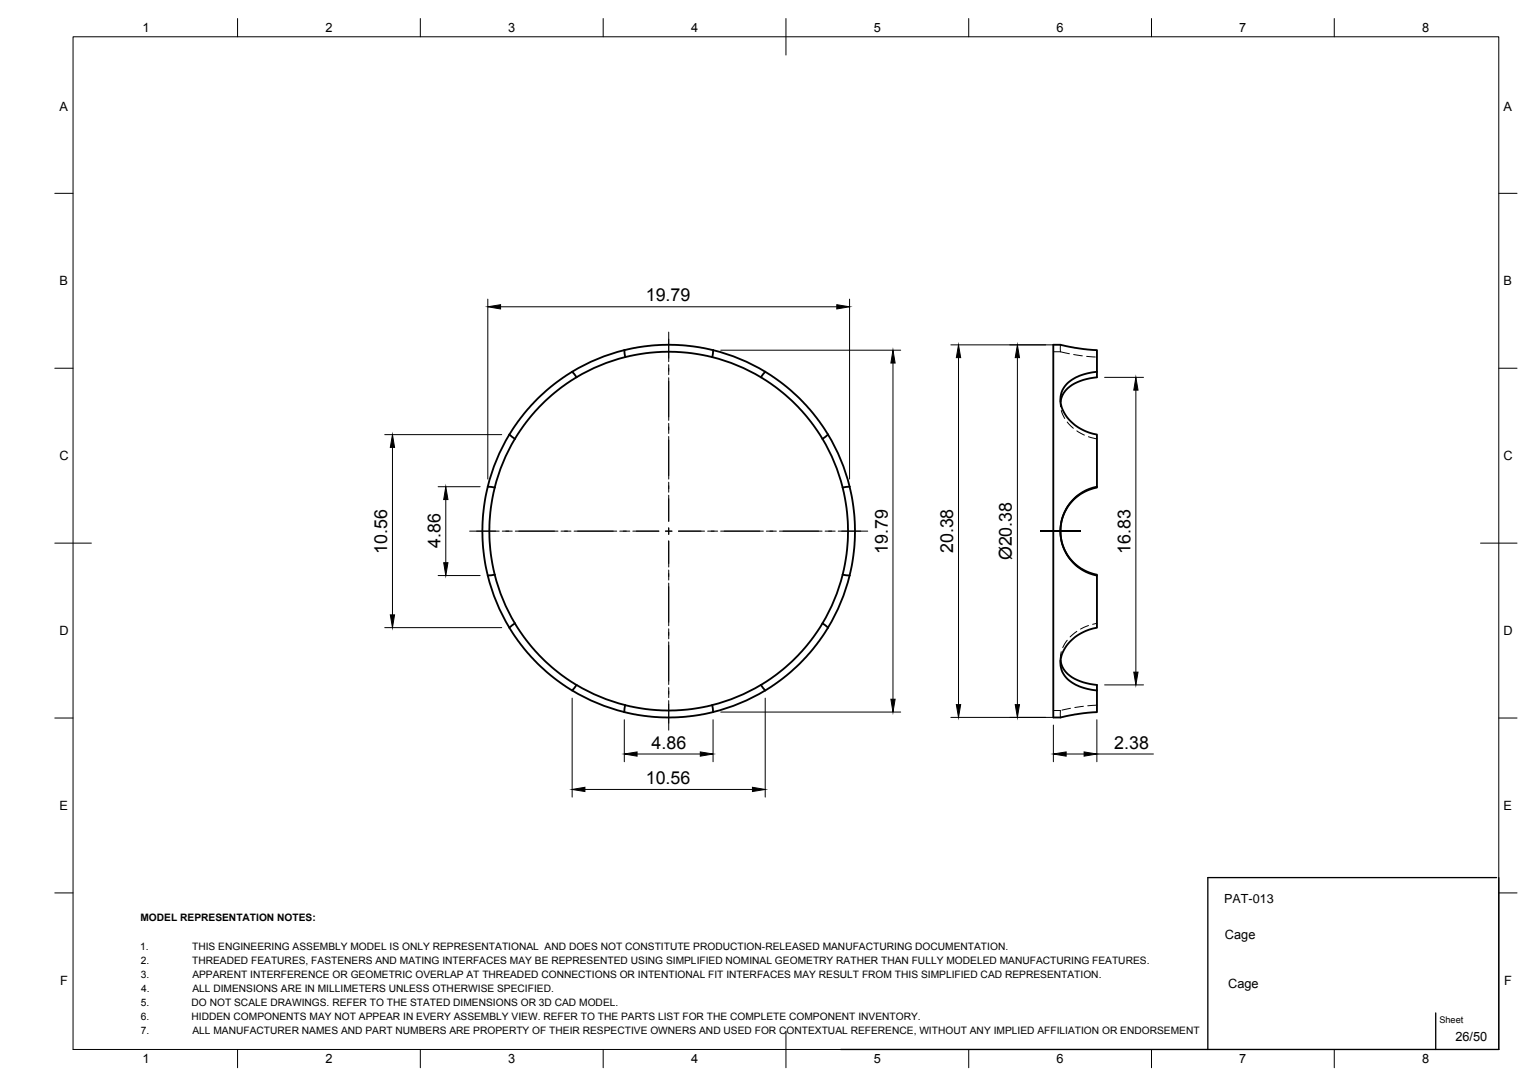
ISO-10303-21;
HEADER;
/* Generated by software containing ST-Developer
 * from STEP Tools, Inc. (www.steptools.com) 
 */

FILE_DESCRIPTION(
/* description */ ('Belt-driven linear axis on 2020 extrusion'),
/* implementation_level */ '2;1');

FILE_NAME(
/* name */ 'Cage.step',
/* time_stamp */ '2026-10-28T03:26:09-07:00',
/* author */ (''),
/* organization */ (''),
/* preprocessor_version */ 'ST-DEVELOPER v20.2',
/* originating_system */ 'Autodesk Translation Framework v15.17.0.0',
/* authorisation */ '');

FILE_SCHEMA (('AUTOMOTIVE_DESIGN { 1 0 10303 214 3 1 1 }'));
ENDSEC;

DATA;
#10=MECHANICAL_DESIGN_GEOMETRIC_PRESENTATION_REPRESENTATION('',(#636),#20096);
#441=B_SPLINE_CURVE_WITH_KNOTS('',3,(#17380,#17381,#17382,#17383,#17384,
#17385,#17386,#17387,#17388,#17389,#17390,#17391,#17392,#17393,#17394,#17395,
#17396,#17397,#17398,#17399,#17400,#17401),.UNSPECIFIED.,.F.,.F.,(4,2,2,
2,2,2,2,2,2,2,4),(0.0473477652366656,0.126350602536658,0.189525903804987,
0.252701205073317,0.313298422430275,0.373895639787233,0.434492857144191,
0.495090074501149,0.558265375769478,0.621440677037807,0.7004435143378),
 .UNSPECIFIED.);
#442=B_SPLINE_CURVE_WITH_KNOTS('',3,(#17405,#17406,#17407,#17408,#17409,
#17410,#17411,#17412,#17413,#17414,#17415,#17416,#17417,#17418,#17419,#17420,
#17421,#17422,#17423,#17424,#17425,#17426),.UNSPECIFIED.,.F.,.F.,(4,2,2,
2,2,2,2,2,2,2,4),(0.0464897534940957,0.0852567806515119,0.170513561303024,
0.246687263103517,0.308657850341199,0.370628437578881,0.432599024816563,
0.494569612054245,0.570743313854739,0.656000094506251,0.694767121663666),
 .UNSPECIFIED.);
#443=B_SPLINE_CURVE_WITH_KNOTS('',3,(#17432,#17433,#17434,#17435,#17436,
#17437,#17438,#17439,#17440,#17441,#17442,#17443,#17444,#17445,#17446,#17447,
#17448,#17449,#17450,#17451,#17452,#17453),.UNSPECIFIED.,.F.,.F.,(4,2,2,
2,2,2,2,2,2,2,4),(0.0464897534940957,0.0852567806515118,0.170513561303024,
0.246687263103517,0.308657850341199,0.370628437578881,0.432599024816563,
0.494569612054245,0.570743313854738,0.65600009450625,0.694767121663666),
 .UNSPECIFIED.);
#444=B_SPLINE_CURVE_WITH_KNOTS('',3,(#17457,#17458,#17459,#17460,#17461,
#17462,#17463,#17464,#17465,#17466,#17467,#17468,#17469,#17470,#17471,#17472,
#17473,#17474,#17475,#17476,#17477,#17478),.UNSPECIFIED.,.F.,.F.,(4,2,2,
2,2,2,2,2,2,2,4),(0.0464897534940957,0.0852567806515119,0.170513561303024,
0.246687263103517,0.308657850341199,0.370628437578881,0.432599024816563,
0.494569612054245,0.570743313854739,0.656000094506251,0.694767121663666),
 .UNSPECIFIED.);
#445=B_SPLINE_CURVE_WITH_KNOTS('',3,(#17482,#17483,#17484,#17485,#17486,
#17487,#17488,#17489,#17490,#17491,#17492,#17493),.UNSPECIFIED.,.F.,.F.,
(4,2,2,2,2,4),(0.0464897534940957,0.0852567806515119,0.170513561303024,
0.246687263103517,0.308657850341199,0.370628437578881),.UNSPECIFIED.);
#446=B_SPLINE_CURVE_WITH_KNOTS('',3,(#17498,#17499,#17500,#17501,#17502,
#17503,#17504,#17505,#17506,#17507,#17508,#17509),.UNSPECIFIED.,.F.,.F.,
(4,2,2,2,2,4),(0.370628437578881,0.432599024816563,0.494569612054245,0.570743313854738,
0.65600009450625,0.694767121663666),.UNSPECIFIED.);
#447=B_SPLINE_CURVE_WITH_KNOTS('',3,(#17513,#17514,#17515,#17516,#17517,
#17518,#17519,#17520,#17521,#17522,#17523,#17524,#17525,#17526,#17527,#17528,
#17529,#17530,#17531,#17532,#17533,#17534),.UNSPECIFIED.,.F.,.F.,(4,2,2,
2,2,2,2,2,2,2,4),(0.0464897534940957,0.0852567806515121,0.170513561303024,
0.246687263103518,0.308657850341199,0.370628437578881,0.432599024816563,
0.494569612054245,0.570743313854738,0.65600009450625,0.694767121663666),
 .UNSPECIFIED.);
#448=B_SPLINE_CURVE_WITH_KNOTS('',3,(#17538,#17539,#17540,#17541,#17542,
#17543,#17544,#17545,#17546,#17547,#17548,#17549,#17550,#17551,#17552,#17553,
#17554,#17555,#17556,#17557,#17558,#17559),.UNSPECIFIED.,.F.,.F.,(4,2,2,
2,2,2,2,2,2,2,4),(0.0464897534940957,0.0852567806515119,0.170513561303024,
0.246687263103517,0.308657850341199,0.370628437578881,0.432599024816563,
0.494569612054245,0.570743313854738,0.65600009450625,0.694767121663667),
 .UNSPECIFIED.);
#449=B_SPLINE_CURVE_WITH_KNOTS('',3,(#17563,#17564,#17565,#17566,#17567,
#17568,#17569,#17570,#17571,#17572,#17573,#17574,#17575,#17576,#17577,#17578,
#17579,#17580,#17581,#17582,#17583,#17584),.UNSPECIFIED.,.F.,.F.,(4,2,2,
2,2,2,2,2,2,2,4),(0.0464897534940957,0.0852567806515119,0.170513561303024,
0.246687263103517,0.308657850341199,0.370628437578881,0.432599024816563,
0.494569612054245,0.570743313854738,0.65600009450625,0.694767121663666),
 .UNSPECIFIED.);
#450=B_SPLINE_CURVE_WITH_KNOTS('',3,(#17588,#17589,#17590,#17591,#17592,
#17593,#17594,#17595,#17596,#17597,#17598,#17599,#17600,#17601,#17602,#17603,
#17604,#17605,#17606,#17607,#17608,#17609),.UNSPECIFIED.,.F.,.F.,(4,2,2,
2,2,2,2,2,2,2,4),(0.0464897534940957,0.0852567806515119,0.170513561303024,
0.246687263103517,0.308657850341199,0.370628437578881,0.432599024816563,
0.494569612054245,0.570743313854739,0.656000094506251,0.694767121663667),
 .UNSPECIFIED.);
#451=B_SPLINE_CURVE_WITH_KNOTS('',3,(#17617,#17618,#17619,#17620,#17621,
#17622,#17623,#17624,#17625,#17626,#17627,#17628,#17629,#17630,#17631,#17632,
#17633,#17634,#17635,#17636,#17637,#17638),.UNSPECIFIED.,.F.,.F.,(4,2,2,
2,2,2,2,2,2,2,4),(0.0473477652366656,0.126350602536658,0.189525903804987,
0.252701205073316,0.313298422430274,0.373895639787232,0.434492857144191,
0.495090074501149,0.558265375769478,0.621440677037807,0.7004435143378),
 .UNSPECIFIED.);
#452=B_SPLINE_CURVE_WITH_KNOTS('',3,(#17646,#17647,#17648,#17649,#17650,
#17651,#17652,#17653,#17654,#17655,#17656,#17657,#17658,#17659,#17660,#17661,
#17662,#17663,#17664,#17665,#17666,#17667),.UNSPECIFIED.,.F.,.F.,(4,2,2,
2,2,2,2,2,2,2,4),(0.0473477652366656,0.126350602536658,0.189525903804987,
0.252701205073317,0.313298422430275,0.373895639787233,0.434492857144191,
0.495090074501149,0.558265375769478,0.621440677037807,0.7004435143378),
 .UNSPECIFIED.);
#453=B_SPLINE_CURVE_WITH_KNOTS('',3,(#17676,#17677,#17678,#17679,#17680,
#17681,#17682,#17683,#17684,#17685,#17686,#17687),.UNSPECIFIED.,.F.,.F.,
(4,2,2,2,2,4),(0.0473477652366656,0.126350602536658,0.189525903804987,0.252701205073316,
0.313298422430275,0.373895639787233),.UNSPECIFIED.);
#454=B_SPLINE_CURVE_WITH_KNOTS('',3,(#17689,#17690,#17691,#17692,#17693,
#17694,#17695,#17696,#17697,#17698,#17699,#17700),.UNSPECIFIED.,.F.,.F.,
(4,2,2,2,2,4),(0.373895639787233,0.434492857144191,0.495090074501149,0.558265375769478,
0.621440677037807,0.7004435143378),.UNSPECIFIED.);
#455=B_SPLINE_CURVE_WITH_KNOTS('',3,(#17707,#17708,#17709,#17710,#17711,
#17712,#17713,#17714,#17715,#17716,#17717,#17718,#17719,#17720,#17721,#17722,
#17723,#17724,#17725,#17726,#17727,#17728),.UNSPECIFIED.,.F.,.F.,(4,2,2,
2,2,2,2,2,2,2,4),(0.0473477652366656,0.126350602536658,0.189525903804987,
0.252701205073316,0.313298422430275,0.373895639787233,0.434492857144191,
0.495090074501149,0.558265375769478,0.621440677037807,0.7004435143378),
 .UNSPECIFIED.);
#456=B_SPLINE_CURVE_WITH_KNOTS('',3,(#17736,#17737,#17738,#17739,#17740,
#17741,#17742,#17743,#17744,#17745,#17746,#17747,#17748,#17749,#17750,#17751,
#17752,#17753,#17754,#17755,#17756,#17757),.UNSPECIFIED.,.F.,.F.,(4,2,2,
2,2,2,2,2,2,2,4),(0.0473477652366656,0.126350602536658,0.189525903804987,
0.252701205073317,0.313298422430275,0.373895639787233,0.434492857144191,
0.495090074501149,0.558265375769478,0.621440677037807,0.7004435143378),
 .UNSPECIFIED.);
#457=B_SPLINE_CURVE_WITH_KNOTS('',3,(#17765,#17766,#17767,#17768,#17769,
#17770,#17771,#17772,#17773,#17774,#17775,#17776,#17777,#17778,#17779,#17780,
#17781,#17782,#17783,#17784,#17785,#17786),.UNSPECIFIED.,.F.,.F.,(4,2,2,
2,2,2,2,2,2,2,4),(0.0473477652366656,0.126350602536658,0.189525903804987,
0.252701205073316,0.313298422430275,0.373895639787233,0.434492857144191,
0.495090074501149,0.558265375769478,0.621440677037807,0.7004435143378),
 .UNSPECIFIED.);
#458=B_SPLINE_CURVE_WITH_KNOTS('',3,(#17795,#17796,#17797,#17798,#17799,
#17800,#17801,#17802,#17803,#17804,#17805,#17806,#17807,#17808,#17809,#17810,
#17811,#17812,#17813,#17814,#17815,#17816),.UNSPECIFIED.,.F.,.F.,(4,2,2,
2,2,2,2,2,2,2,4),(0.0473477652366656,0.126350602536658,0.189525903804987,
0.252701205073317,0.313298422430275,0.373895639787233,0.434492857144191,
0.495090074501149,0.558265375769478,0.621440677037807,0.7004435143378),
 .UNSPECIFIED.);
#489=SPHERICAL_SURFACE('',#11975,0.247676);
#490=SPHERICAL_SURFACE('',#11991,0.247676);
#491=SPHERICAL_SURFACE('',#11996,0.247676);
#492=SPHERICAL_SURFACE('',#12001,0.247676);
#493=SPHERICAL_SURFACE('',#12006,0.247676);
#494=SPHERICAL_SURFACE('',#12011,0.247676);
#495=SPHERICAL_SURFACE('',#12016,0.247676);
#496=SPHERICAL_SURFACE('',#12024,0.247676);
#535=SHAPE_REPRESENTATION_RELATIONSHIP('SRR','None',#20332,#581);
#581=ADVANCED_BREP_SHAPE_REPRESENTATION('',(#692),#20063);
#636=STYLED_ITEM('',(#20650),#692);
#692=MANIFOLD_SOLID_BREP('Continuous crown cage',#10949);
#808=FACE_BOUND('',#2218,.T.);
#1009=PLANE('',#11988);
#1010=PLANE('',#11993);
#1011=PLANE('',#11998);
#1012=PLANE('',#12003);
#1013=PLANE('',#12008);
#1014=PLANE('',#12013);
#1015=PLANE('',#12022);
#1016=PLANE('',#12026);
#1017=PLANE('',#12027);
#1488=FACE_OUTER_BOUND('',#2200,.T.);
#1489=FACE_OUTER_BOUND('',#2201,.T.);
#1490=FACE_OUTER_BOUND('',#2202,.T.);
#1491=FACE_OUTER_BOUND('',#2203,.T.);
#1492=FACE_OUTER_BOUND('',#2204,.T.);
#1493=FACE_OUTER_BOUND('',#2205,.T.);
#1494=FACE_OUTER_BOUND('',#2206,.T.);
#1495=FACE_OUTER_BOUND('',#2207,.T.);
#1496=FACE_OUTER_BOUND('',#2208,.T.);
#1497=FACE_OUTER_BOUND('',#2209,.T.);
#1498=FACE_OUTER_BOUND('',#2210,.T.);
#1499=FACE_OUTER_BOUND('',#2211,.T.);
#1500=FACE_OUTER_BOUND('',#2212,.T.);
#1501=FACE_OUTER_BOUND('',#2213,.T.);
#1502=FACE_OUTER_BOUND('',#2214,.T.);
#1503=FACE_OUTER_BOUND('',#2215,.T.);
#1504=FACE_OUTER_BOUND('',#2216,.T.);
#1505=FACE_OUTER_BOUND('',#2217,.T.);
#1506=FACE_OUTER_BOUND('',#2219,.T.);
#2200=EDGE_LOOP('',(#8305,#8306,#8307,#8308));
#2201=EDGE_LOOP('',(#8309,#8310,#8311,#8312,#8313,#8314,#8315,#8316,#8317,
#8318,#8319,#8320,#8321,#8322,#8323,#8324,#8325,#8326,#8327,#8328));
#2202=EDGE_LOOP('',(#8329,#8330,#8331,#8332));
#2203=EDGE_LOOP('',(#8333,#8334,#8335,#8336));
#2204=EDGE_LOOP('',(#8337,#8338,#8339,#8340));
#2205=EDGE_LOOP('',(#8341,#8342,#8343,#8344));
#2206=EDGE_LOOP('',(#8345,#8346,#8347,#8348));
#2207=EDGE_LOOP('',(#8349,#8350,#8351,#8352,#8353,#8354));
#2208=EDGE_LOOP('',(#8355,#8356,#8357,#8358));
#2209=EDGE_LOOP('',(#8359,#8360,#8361,#8362));
#2210=EDGE_LOOP('',(#8363,#8364,#8365,#8366));
#2211=EDGE_LOOP('',(#8367,#8368,#8369,#8370));
#2212=EDGE_LOOP('',(#8371,#8372,#8373,#8374));
#2213=EDGE_LOOP('',(#8375,#8376,#8377,#8378));
#2214=EDGE_LOOP('',(#8379,#8380,#8381,#8382,#8383,#8384,#8385,#8386,#8387,
#8388,#8389,#8390,#8391,#8392,#8393,#8394,#8395,#8396,#8397,#8398));
#2215=EDGE_LOOP('',(#8399,#8400,#8401,#8402));
#2216=EDGE_LOOP('',(#8403,#8404,#8405,#8406));
#2217=EDGE_LOOP('',(#8407));
#2218=EDGE_LOOP('',(#8408));
#2219=EDGE_LOOP('',(#8409,#8410,#8411,#8412));
#2965=LINE('',#17495,#3822);
#2966=LINE('',#17791,#3823);
#3822=VECTOR('',#14069,1.019052);
#3823=VECTOR('',#14146,0.980948);
#4605=CIRCLE('',#11976,0.243053047864041);
#4606=CIRCLE('',#11977,0.243053047864041);
#4607=CIRCLE('',#11979,1.019052);
#4608=CIRCLE('',#11980,1.019052);
#4609=CIRCLE('',#11981,1.019052);
#4610=CIRCLE('',#11982,1.019052);
#4611=CIRCLE('',#11983,1.019052);
#4612=CIRCLE('',#11984,1.019052);
#4613=CIRCLE('',#11985,1.019052);
#4614=CIRCLE('',#11986,1.019052);
#4615=CIRCLE('',#11987,1.019052);
#4616=CIRCLE('',#11989,0.980948);
#4617=CIRCLE('',#11990,0.243053047864041);
#4618=CIRCLE('',#11992,0.243053047864041);
#4619=CIRCLE('',#11994,0.980948);
#4620=CIRCLE('',#11995,0.243053047864041);
#4621=CIRCLE('',#11997,0.243053047864041);
#4622=CIRCLE('',#11999,0.980948);
#4623=CIRCLE('',#12000,0.243053047864041);
#4624=CIRCLE('',#12002,0.243053047864041);
#4625=CIRCLE('',#12004,0.980948);
#4626=CIRCLE('',#12005,0.243053047864041);
#4627=CIRCLE('',#12007,0.243053047864041);
#4628=CIRCLE('',#12009,0.980948);
#4629=CIRCLE('',#12010,0.243053047864041);
#4630=CIRCLE('',#12012,0.243053047864041);
#4631=CIRCLE('',#12014,0.980948);
#4632=CIRCLE('',#12015,0.243053047864041);
#4633=CIRCLE('',#12017,0.243053047864041);
#4634=CIRCLE('',#12019,0.980948);
#4635=CIRCLE('',#12020,0.980948);
#4636=CIRCLE('',#12021,0.980948);
#4637=CIRCLE('',#12023,0.243053047864041);
#4638=CIRCLE('',#12025,0.243053047864041);
#5252=VERTEX_POINT('',#17378);
#5253=VERTEX_POINT('',#17379);
#5254=VERTEX_POINT('',#17402);
#5255=VERTEX_POINT('',#17404);
#5256=VERTEX_POINT('',#17429);
#5257=VERTEX_POINT('',#17431);
#5258=VERTEX_POINT('',#17454);
#5259=VERTEX_POINT('',#17456);
#5260=VERTEX_POINT('',#17479);
#5261=VERTEX_POINT('',#17481);
#5262=VERTEX_POINT('',#17494);
#5263=VERTEX_POINT('',#17497);
#5264=VERTEX_POINT('',#17510);
#5265=VERTEX_POINT('',#17512);
#5266=VERTEX_POINT('',#17535);
#5267=VERTEX_POINT('',#17537);
#5268=VERTEX_POINT('',#17560);
#5269=VERTEX_POINT('',#17562);
#5270=VERTEX_POINT('',#17585);
#5271=VERTEX_POINT('',#17587);
#5272=VERTEX_POINT('',#17612);
#5273=VERTEX_POINT('',#17616);
#5274=VERTEX_POINT('',#17641);
#5275=VERTEX_POINT('',#17645);
#5276=VERTEX_POINT('',#17670);
#5277=VERTEX_POINT('',#17674);
#5278=VERTEX_POINT('',#17675);
#5279=VERTEX_POINT('',#17702);
#5280=VERTEX_POINT('',#17706);
#5281=VERTEX_POINT('',#17731);
#5282=VERTEX_POINT('',#17735);
#5283=VERTEX_POINT('',#17760);
#5284=VERTEX_POINT('',#17764);
#5285=VERTEX_POINT('',#17789);
#5286=VERTEX_POINT('',#17792);
#5287=VERTEX_POINT('',#17794);
#6367=EDGE_CURVE('',#5252,#5253,#441,.T.);
#6368=EDGE_CURVE('',#5254,#5252,#4605,.T.);
#6369=EDGE_CURVE('',#5255,#5254,#442,.T.);
#6370=EDGE_CURVE('',#5253,#5255,#4606,.T.);
#6371=EDGE_CURVE('',#5256,#5254,#4607,.T.);
#6372=EDGE_CURVE('',#5256,#5257,#443,.T.);
#6373=EDGE_CURVE('',#5258,#5257,#4608,.T.);
#6374=EDGE_CURVE('',#5258,#5259,#444,.T.);
#6375=EDGE_CURVE('',#5260,#5259,#4609,.T.);
#6376=EDGE_CURVE('',#5260,#5261,#445,.T.);
#6377=EDGE_CURVE('',#5261,#5262,#2965,.T.);
#6378=EDGE_CURVE('',#5262,#5262,#4610,.T.);
#6379=EDGE_CURVE('',#5261,#5263,#446,.T.);
#6380=EDGE_CURVE('',#5264,#5263,#4611,.T.);
#6381=EDGE_CURVE('',#5264,#5265,#447,.T.);
#6382=EDGE_CURVE('',#5266,#5265,#4612,.T.);
#6383=EDGE_CURVE('',#5266,#5267,#448,.T.);
#6384=EDGE_CURVE('',#5268,#5267,#4613,.T.);
#6385=EDGE_CURVE('',#5268,#5269,#449,.T.);
#6386=EDGE_CURVE('',#5270,#5269,#4614,.T.);
#6387=EDGE_CURVE('',#5270,#5271,#450,.T.);
#6388=EDGE_CURVE('',#5255,#5271,#4615,.T.);
#6389=EDGE_CURVE('',#5252,#5272,#4616,.T.);
#6390=EDGE_CURVE('',#5272,#5256,#4617,.T.);
#6391=EDGE_CURVE('',#5273,#5272,#451,.T.);
#6392=EDGE_CURVE('',#5257,#5273,#4618,.T.);
#6393=EDGE_CURVE('',#5273,#5274,#4619,.T.);
#6394=EDGE_CURVE('',#5274,#5258,#4620,.T.);
#6395=EDGE_CURVE('',#5275,#5274,#452,.T.);
#6396=EDGE_CURVE('',#5259,#5275,#4621,.T.);
#6397=EDGE_CURVE('',#5275,#5276,#4622,.T.);
#6398=EDGE_CURVE('',#5276,#5260,#4623,.T.);
#6399=EDGE_CURVE('',#5277,#5278,#453,.T.);
#6400=EDGE_CURVE('',#5263,#5277,#4624,.T.);
#6401=EDGE_CURVE('',#5278,#5276,#454,.T.);
#6402=EDGE_CURVE('',#5277,#5279,#4625,.T.);
#6403=EDGE_CURVE('',#5279,#5264,#4626,.T.);
#6404=EDGE_CURVE('',#5280,#5279,#455,.T.);
#6405=EDGE_CURVE('',#5265,#5280,#4627,.T.);
#6406=EDGE_CURVE('',#5280,#5281,#4628,.T.);
#6407=EDGE_CURVE('',#5281,#5266,#4629,.T.);
#6408=EDGE_CURVE('',#5282,#5281,#456,.T.);
#6409=EDGE_CURVE('',#5267,#5282,#4630,.T.);
#6410=EDGE_CURVE('',#5282,#5283,#4631,.T.);
#6411=EDGE_CURVE('',#5283,#5268,#4632,.T.);
#6412=EDGE_CURVE('',#5284,#5283,#457,.T.);
#6413=EDGE_CURVE('',#5269,#5284,#4633,.T.);
#6414=EDGE_CURVE('',#5285,#5285,#4634,.T.);
#6415=EDGE_CURVE('',#5285,#5278,#2966,.T.);
#6416=EDGE_CURVE('',#5286,#5253,#4635,.T.);
#6417=EDGE_CURVE('',#5286,#5287,#458,.T.);
#6418=EDGE_CURVE('',#5284,#5287,#4636,.T.);
#6419=EDGE_CURVE('',#5271,#5286,#4637,.T.);
#6420=EDGE_CURVE('',#5287,#5270,#4638,.T.);
#8305=ORIENTED_EDGE('',*,*,#6367,.F.);
#8306=ORIENTED_EDGE('',*,*,#6368,.F.);
#8307=ORIENTED_EDGE('',*,*,#6369,.F.);
#8308=ORIENTED_EDGE('',*,*,#6370,.F.);
#8309=ORIENTED_EDGE('',*,*,#6369,.T.);
#8310=ORIENTED_EDGE('',*,*,#6371,.F.);
#8311=ORIENTED_EDGE('',*,*,#6372,.T.);
#8312=ORIENTED_EDGE('',*,*,#6373,.F.);
#8313=ORIENTED_EDGE('',*,*,#6374,.T.);
#8314=ORIENTED_EDGE('',*,*,#6375,.F.);
#8315=ORIENTED_EDGE('',*,*,#6376,.T.);
#8316=ORIENTED_EDGE('',*,*,#6377,.T.);
#8317=ORIENTED_EDGE('',*,*,#6378,.F.);
#8318=ORIENTED_EDGE('',*,*,#6377,.F.);
#8319=ORIENTED_EDGE('',*,*,#6379,.T.);
#8320=ORIENTED_EDGE('',*,*,#6380,.F.);
#8321=ORIENTED_EDGE('',*,*,#6381,.T.);
#8322=ORIENTED_EDGE('',*,*,#6382,.F.);
#8323=ORIENTED_EDGE('',*,*,#6383,.T.);
#8324=ORIENTED_EDGE('',*,*,#6384,.F.);
#8325=ORIENTED_EDGE('',*,*,#6385,.T.);
#8326=ORIENTED_EDGE('',*,*,#6386,.F.);
#8327=ORIENTED_EDGE('',*,*,#6387,.T.);
#8328=ORIENTED_EDGE('',*,*,#6388,.F.);
#8329=ORIENTED_EDGE('',*,*,#6368,.T.);
#8330=ORIENTED_EDGE('',*,*,#6389,.T.);
#8331=ORIENTED_EDGE('',*,*,#6390,.T.);
#8332=ORIENTED_EDGE('',*,*,#6371,.T.);
#8333=ORIENTED_EDGE('',*,*,#6391,.F.);
#8334=ORIENTED_EDGE('',*,*,#6392,.F.);
#8335=ORIENTED_EDGE('',*,*,#6372,.F.);
#8336=ORIENTED_EDGE('',*,*,#6390,.F.);
#8337=ORIENTED_EDGE('',*,*,#6392,.T.);
#8338=ORIENTED_EDGE('',*,*,#6393,.T.);
#8339=ORIENTED_EDGE('',*,*,#6394,.T.);
#8340=ORIENTED_EDGE('',*,*,#6373,.T.);
#8341=ORIENTED_EDGE('',*,*,#6395,.F.);
#8342=ORIENTED_EDGE('',*,*,#6396,.F.);
#8343=ORIENTED_EDGE('',*,*,#6374,.F.);
#8344=ORIENTED_EDGE('',*,*,#6394,.F.);
#8345=ORIENTED_EDGE('',*,*,#6396,.T.);
#8346=ORIENTED_EDGE('',*,*,#6397,.T.);
#8347=ORIENTED_EDGE('',*,*,#6398,.T.);
#8348=ORIENTED_EDGE('',*,*,#6375,.T.);
#8349=ORIENTED_EDGE('',*,*,#6399,.F.);
#8350=ORIENTED_EDGE('',*,*,#6400,.F.);
#8351=ORIENTED_EDGE('',*,*,#6379,.F.);
#8352=ORIENTED_EDGE('',*,*,#6376,.F.);
#8353=ORIENTED_EDGE('',*,*,#6398,.F.);
#8354=ORIENTED_EDGE('',*,*,#6401,.F.);
#8355=ORIENTED_EDGE('',*,*,#6400,.T.);
#8356=ORIENTED_EDGE('',*,*,#6402,.T.);
#8357=ORIENTED_EDGE('',*,*,#6403,.T.);
#8358=ORIENTED_EDGE('',*,*,#6380,.T.);
#8359=ORIENTED_EDGE('',*,*,#6404,.F.);
#8360=ORIENTED_EDGE('',*,*,#6405,.F.);
#8361=ORIENTED_EDGE('',*,*,#6381,.F.);
#8362=ORIENTED_EDGE('',*,*,#6403,.F.);
#8363=ORIENTED_EDGE('',*,*,#6405,.T.);
#8364=ORIENTED_EDGE('',*,*,#6406,.T.);
#8365=ORIENTED_EDGE('',*,*,#6407,.T.);
#8366=ORIENTED_EDGE('',*,*,#6382,.T.);
#8367=ORIENTED_EDGE('',*,*,#6408,.F.);
#8368=ORIENTED_EDGE('',*,*,#6409,.F.);
#8369=ORIENTED_EDGE('',*,*,#6383,.F.);
#8370=ORIENTED_EDGE('',*,*,#6407,.F.);
#8371=ORIENTED_EDGE('',*,*,#6409,.T.);
#8372=ORIENTED_EDGE('',*,*,#6410,.T.);
#8373=ORIENTED_EDGE('',*,*,#6411,.T.);
#8374=ORIENTED_EDGE('',*,*,#6384,.T.);
#8375=ORIENTED_EDGE('',*,*,#6385,.F.);
#8376=ORIENTED_EDGE('',*,*,#6411,.F.);
#8377=ORIENTED_EDGE('',*,*,#6412,.F.);
#8378=ORIENTED_EDGE('',*,*,#6413,.F.);
#8379=ORIENTED_EDGE('',*,*,#6414,.F.);
#8380=ORIENTED_EDGE('',*,*,#6415,.T.);
#8381=ORIENTED_EDGE('',*,*,#6401,.T.);
#8382=ORIENTED_EDGE('',*,*,#6397,.F.);
#8383=ORIENTED_EDGE('',*,*,#6395,.T.);
#8384=ORIENTED_EDGE('',*,*,#6393,.F.);
#8385=ORIENTED_EDGE('',*,*,#6391,.T.);
#8386=ORIENTED_EDGE('',*,*,#6389,.F.);
#8387=ORIENTED_EDGE('',*,*,#6367,.T.);
#8388=ORIENTED_EDGE('',*,*,#6416,.F.);
#8389=ORIENTED_EDGE('',*,*,#6417,.T.);
#8390=ORIENTED_EDGE('',*,*,#6418,.F.);
#8391=ORIENTED_EDGE('',*,*,#6412,.T.);
#8392=ORIENTED_EDGE('',*,*,#6410,.F.);
#8393=ORIENTED_EDGE('',*,*,#6408,.T.);
#8394=ORIENTED_EDGE('',*,*,#6406,.F.);
#8395=ORIENTED_EDGE('',*,*,#6404,.T.);
#8396=ORIENTED_EDGE('',*,*,#6402,.F.);
#8397=ORIENTED_EDGE('',*,*,#6399,.T.);
#8398=ORIENTED_EDGE('',*,*,#6415,.F.);
#8399=ORIENTED_EDGE('',*,*,#6370,.T.);
#8400=ORIENTED_EDGE('',*,*,#6388,.T.);
#8401=ORIENTED_EDGE('',*,*,#6419,.T.);
#8402=ORIENTED_EDGE('',*,*,#6416,.T.);
#8403=ORIENTED_EDGE('',*,*,#6387,.F.);
#8404=ORIENTED_EDGE('',*,*,#6420,.F.);
#8405=ORIENTED_EDGE('',*,*,#6417,.F.);
#8406=ORIENTED_EDGE('',*,*,#6419,.F.);
#8407=ORIENTED_EDGE('',*,*,#6378,.T.);
#8408=ORIENTED_EDGE('',*,*,#6414,.T.);
#8409=ORIENTED_EDGE('',*,*,#6413,.T.);
#8410=ORIENTED_EDGE('',*,*,#6418,.T.);
#8411=ORIENTED_EDGE('',*,*,#6420,.T.);
#8412=ORIENTED_EDGE('',*,*,#6386,.T.);
#10181=CYLINDRICAL_SURFACE('',#11978,1.019052);
#10182=CYLINDRICAL_SURFACE('',#12018,0.980948);
#10539=ADVANCED_FACE('',(#1488),#489,.F.);
#10540=ADVANCED_FACE('',(#1489),#10181,.T.);
#10541=ADVANCED_FACE('',(#1490),#1009,.T.);
#10542=ADVANCED_FACE('',(#1491),#490,.F.);
#10543=ADVANCED_FACE('',(#1492),#1010,.T.);
#10544=ADVANCED_FACE('',(#1493),#491,.F.);
#10545=ADVANCED_FACE('',(#1494),#1011,.T.);
#10546=ADVANCED_FACE('',(#1495),#492,.F.);
#10547=ADVANCED_FACE('',(#1496),#1012,.T.);
#10548=ADVANCED_FACE('',(#1497),#493,.F.);
#10549=ADVANCED_FACE('',(#1498),#1013,.T.);
#10550=ADVANCED_FACE('',(#1499),#494,.F.);
#10551=ADVANCED_FACE('',(#1500),#1014,.T.);
#10552=ADVANCED_FACE('',(#1501),#495,.F.);
#10553=ADVANCED_FACE('',(#1502),#10182,.F.);
#10554=ADVANCED_FACE('',(#1503),#1015,.T.);
#10555=ADVANCED_FACE('',(#1504),#496,.F.);
#10556=ADVANCED_FACE('',(#1505,#808),#1016,.T.);
#10557=ADVANCED_FACE('',(#1506),#1017,.T.);
#10949=CLOSED_SHELL('',(#10539,#10540,#10541,#10542,#10543,#10544,#10545,
#10546,#10547,#10548,#10549,#10550,#10551,#10552,#10553,#10554,#10555,#10556,
#10557));
#11974=AXIS2_PLACEMENT_3D('',#17376,#14053,#14054);
#11975=AXIS2_PLACEMENT_3D('',#17377,#14055,#14056);
#11976=AXIS2_PLACEMENT_3D('',#17403,#14057,#14058);
#11977=AXIS2_PLACEMENT_3D('',#17427,#14059,#14060);
#11978=AXIS2_PLACEMENT_3D('',#17428,#14061,#14062);
#11979=AXIS2_PLACEMENT_3D('',#17430,#14063,#14064);
#11980=AXIS2_PLACEMENT_3D('',#17455,#14065,#14066);
#11981=AXIS2_PLACEMENT_3D('',#17480,#14067,#14068);
#11982=AXIS2_PLACEMENT_3D('',#17496,#14070,#14071);
#11983=AXIS2_PLACEMENT_3D('',#17511,#14072,#14073);
#11984=AXIS2_PLACEMENT_3D('',#17536,#14074,#14075);
#11985=AXIS2_PLACEMENT_3D('',#17561,#14076,#14077);
#11986=AXIS2_PLACEMENT_3D('',#17586,#14078,#14079);
#11987=AXIS2_PLACEMENT_3D('',#17610,#14080,#14081);
#11988=AXIS2_PLACEMENT_3D('',#17611,#14082,#14083);
#11989=AXIS2_PLACEMENT_3D('',#17613,#14084,#14085);
#11990=AXIS2_PLACEMENT_3D('',#17614,#14086,#14087);
#11991=AXIS2_PLACEMENT_3D('',#17615,#14088,#14089);
#11992=AXIS2_PLACEMENT_3D('',#17639,#14090,#14091);
#11993=AXIS2_PLACEMENT_3D('',#17640,#14092,#14093);
#11994=AXIS2_PLACEMENT_3D('',#17642,#14094,#14095);
#11995=AXIS2_PLACEMENT_3D('',#17643,#14096,#14097);
#11996=AXIS2_PLACEMENT_3D('',#17644,#14098,#14099);
#11997=AXIS2_PLACEMENT_3D('',#17668,#14100,#14101);
#11998=AXIS2_PLACEMENT_3D('',#17669,#14102,#14103);
#11999=AXIS2_PLACEMENT_3D('',#17671,#14104,#14105);
#12000=AXIS2_PLACEMENT_3D('',#17672,#14106,#14107);
#12001=AXIS2_PLACEMENT_3D('',#17673,#14108,#14109);
#12002=AXIS2_PLACEMENT_3D('',#17688,#14110,#14111);
#12003=AXIS2_PLACEMENT_3D('',#17701,#14112,#14113);
#12004=AXIS2_PLACEMENT_3D('',#17703,#14114,#14115);
#12005=AXIS2_PLACEMENT_3D('',#17704,#14116,#14117);
#12006=AXIS2_PLACEMENT_3D('',#17705,#14118,#14119);
#12007=AXIS2_PLACEMENT_3D('',#17729,#14120,#14121);
#12008=AXIS2_PLACEMENT_3D('',#17730,#14122,#14123);
#12009=AXIS2_PLACEMENT_3D('',#17732,#14124,#14125);
#12010=AXIS2_PLACEMENT_3D('',#17733,#14126,#14127);
#12011=AXIS2_PLACEMENT_3D('',#17734,#14128,#14129);
#12012=AXIS2_PLACEMENT_3D('',#17758,#14130,#14131);
#12013=AXIS2_PLACEMENT_3D('',#17759,#14132,#14133);
#12014=AXIS2_PLACEMENT_3D('',#17761,#14134,#14135);
#12015=AXIS2_PLACEMENT_3D('',#17762,#14136,#14137);
#12016=AXIS2_PLACEMENT_3D('',#17763,#14138,#14139);
#12017=AXIS2_PLACEMENT_3D('',#17787,#14140,#14141);
#12018=AXIS2_PLACEMENT_3D('',#17788,#14142,#14143);
#12019=AXIS2_PLACEMENT_3D('',#17790,#14144,#14145);
#12020=AXIS2_PLACEMENT_3D('',#17793,#14147,#14148);
#12021=AXIS2_PLACEMENT_3D('',#17817,#14149,#14150);
#12022=AXIS2_PLACEMENT_3D('',#17818,#14151,#14152);
#12023=AXIS2_PLACEMENT_3D('',#17819,#14153,#14154);
#12024=AXIS2_PLACEMENT_3D('',#17820,#14155,#14156);
#12025=AXIS2_PLACEMENT_3D('',#17821,#14157,#14158);
#12026=AXIS2_PLACEMENT_3D('',#17822,#14159,#14160);
#12027=AXIS2_PLACEMENT_3D('',#17823,#14161,#14162);
#14053=DIRECTION('axis',(0.,0.,1.));
#14054=DIRECTION('refdir',(1.,0.,0.));
#14055=DIRECTION('center_axis',(0.,0.,1.));
#14056=DIRECTION('ref_axis',(1.,0.,0.));
#14057=DIRECTION('center_axis',(0.,-1.,0.));
#14058=DIRECTION('ref_axis',(0.,0.,-1.));
#14059=DIRECTION('center_axis',(0.,-1.,0.));
#14060=DIRECTION('ref_axis',(0.,0.,-1.));
#14061=DIRECTION('center_axis',(0.,1.,0.));
#14062=DIRECTION('ref_axis',(1.,0.,0.));
#14063=DIRECTION('center_axis',(0.,1.,0.));
#14064=DIRECTION('ref_axis',(1.,0.,0.));
#14065=DIRECTION('center_axis',(0.,1.,0.));
#14066=DIRECTION('ref_axis',(1.,0.,0.));
#14067=DIRECTION('center_axis',(0.,1.,0.));
#14068=DIRECTION('ref_axis',(1.,0.,0.));
#14069=DIRECTION('',(0.,-1.,0.));
#14070=DIRECTION('center_axis',(0.,-1.,0.));
#14071=DIRECTION('ref_axis',(1.,0.,0.));
#14072=DIRECTION('center_axis',(0.,1.,0.));
#14073=DIRECTION('ref_axis',(1.,0.,0.));
#14074=DIRECTION('center_axis',(0.,1.,0.));
#14075=DIRECTION('ref_axis',(1.,0.,0.));
#14076=DIRECTION('center_axis',(0.,1.,0.));
#14077=DIRECTION('ref_axis',(1.,0.,0.));
#14078=DIRECTION('center_axis',(0.,1.,0.));
#14079=DIRECTION('ref_axis',(1.,0.,0.));
#14080=DIRECTION('center_axis',(0.,1.,0.));
#14081=DIRECTION('ref_axis',(1.,0.,0.));
#14082=DIRECTION('center_axis',(0.,1.,0.));
#14083=DIRECTION('ref_axis',(1.,0.,0.));
#14084=DIRECTION('center_axis',(0.,-1.,0.));
#14085=DIRECTION('ref_axis',(1.,0.,0.));
#14086=DIRECTION('center_axis',(0.,-1.,0.));
#14087=DIRECTION('ref_axis',(0.,0.,-1.));
#14088=DIRECTION('center_axis',(6.12323399573677E-17,0.,1.));
#14089=DIRECTION('ref_axis',(1.,0.,0.));
#14090=DIRECTION('center_axis',(0.,-1.,0.));
#14091=DIRECTION('ref_axis',(0.,0.,-1.));
#14092=DIRECTION('center_axis',(0.,1.,0.));
#14093=DIRECTION('ref_axis',(1.,0.,0.));
#14094=DIRECTION('center_axis',(0.,-1.,0.));
#14095=DIRECTION('ref_axis',(1.,0.,0.));
#14096=DIRECTION('center_axis',(0.,-1.,0.));
#14097=DIRECTION('ref_axis',(0.,0.,-1.));
#14098=DIRECTION('center_axis',(0.,0.,1.));
#14099=DIRECTION('ref_axis',(1.,0.,0.));
#14100=DIRECTION('center_axis',(0.,-1.,0.));
#14101=DIRECTION('ref_axis',(0.,0.,-1.));
#14102=DIRECTION('center_axis',(0.,1.,0.));
#14103=DIRECTION('ref_axis',(1.,0.,0.));
#14104=DIRECTION('center_axis',(0.,-1.,0.));
#14105=DIRECTION('ref_axis',(1.,0.,0.));
#14106=DIRECTION('center_axis',(0.,-1.,0.));
#14107=DIRECTION('ref_axis',(0.,0.,-1.));
#14108=DIRECTION('center_axis',(0.,0.,1.));
#14109=DIRECTION('ref_axis',(1.,0.,0.));
#14110=DIRECTION('center_axis',(0.,-1.,0.));
#14111=DIRECTION('ref_axis',(0.,0.,-1.));
#14112=DIRECTION('center_axis',(0.,1.,0.));
#14113=DIRECTION('ref_axis',(1.,0.,0.));
#14114=DIRECTION('center_axis',(0.,-1.,0.));
#14115=DIRECTION('ref_axis',(1.,0.,0.));
#14116=DIRECTION('center_axis',(0.,-1.,0.));
#14117=DIRECTION('ref_axis',(0.,0.,-1.));
#14118=DIRECTION('center_axis',(0.,0.,1.));
#14119=DIRECTION('ref_axis',(1.,0.,0.));
#14120=DIRECTION('center_axis',(0.,-1.,0.));
#14121=DIRECTION('ref_axis',(0.,0.,-1.));
#14122=DIRECTION('center_axis',(0.,1.,0.));
#14123=DIRECTION('ref_axis',(1.,0.,0.));
#14124=DIRECTION('center_axis',(0.,-1.,0.));
#14125=DIRECTION('ref_axis',(1.,0.,0.));
#14126=DIRECTION('center_axis',(0.,-1.,0.));
#14127=DIRECTION('ref_axis',(0.,0.,-1.));
#14128=DIRECTION('center_axis',(6.12323399573676E-17,0.,1.));
#14129=DIRECTION('ref_axis',(1.,0.,0.));
#14130=DIRECTION('center_axis',(0.,-1.,0.));
#14131=DIRECTION('ref_axis',(0.,0.,-1.));
#14132=DIRECTION('center_axis',(0.,1.,0.));
#14133=DIRECTION('ref_axis',(1.,0.,0.));
#14134=DIRECTION('center_axis',(0.,-1.,0.));
#14135=DIRECTION('ref_axis',(1.,0.,0.));
#14136=DIRECTION('center_axis',(0.,-1.,0.));
#14137=DIRECTION('ref_axis',(0.,0.,-1.));
#14138=DIRECTION('center_axis',(0.,0.,1.));
#14139=DIRECTION('ref_axis',(1.,0.,0.));
#14140=DIRECTION('center_axis',(0.,-1.,0.));
#14141=DIRECTION('ref_axis',(0.,0.,-1.));
#14142=DIRECTION('center_axis',(0.,1.,0.));
#14143=DIRECTION('ref_axis',(1.,0.,0.));
#14144=DIRECTION('center_axis',(0.,1.,0.));
#14145=DIRECTION('ref_axis',(1.,0.,0.));
#14146=DIRECTION('',(0.,1.,0.));
#14147=DIRECTION('center_axis',(0.,-1.,0.));
#14148=DIRECTION('ref_axis',(1.,0.,0.));
#14149=DIRECTION('center_axis',(0.,-1.,0.));
#14150=DIRECTION('ref_axis',(1.,0.,0.));
#14151=DIRECTION('center_axis',(0.,1.,0.));
#14152=DIRECTION('ref_axis',(1.,0.,0.));
#14153=DIRECTION('center_axis',(0.,-1.,0.));
#14154=DIRECTION('ref_axis',(0.,0.,-1.));
#14155=DIRECTION('center_axis',(0.,0.,1.));
#14156=DIRECTION('ref_axis',(1.,0.,0.));
#14157=DIRECTION('center_axis',(0.,-1.,0.));
#14158=DIRECTION('ref_axis',(0.,0.,-1.));
#14159=DIRECTION('center_axis',(0.,-1.,0.));
#14160=DIRECTION('ref_axis',(-1.,0.,0.));
#14161=DIRECTION('center_axis',(0.,1.,0.));
#14162=DIRECTION('ref_axis',(1.,0.,0.));
#17376=CARTESIAN_POINT('',(0.,0.,0.));
#17377=CARTESIAN_POINT('Origin',(0.707106781186547,0.,0.707106781186548));
#17378=CARTESIAN_POINT('',(0.504455939115715,-0.04763,0.841298510752802));
#17379=CARTESIAN_POINT('',(0.841298510752802,-0.04763,0.504455939115715));
#17380=CARTESIAN_POINT('Ctrl Pts',(0.504455939115715,-0.04763,0.841298510752802));
#17381=CARTESIAN_POINT('Ctrl Pts',(0.508899795931835,-0.0740444353928835,
0.838633903678357));
#17382=CARTESIAN_POINT('Ctrl Pts',(0.517157748491652,-0.0999305678883309,
0.833661031856294));
#17383=CARTESIAN_POINT('Ctrl Pts',(0.537715343527944,-0.142345102874864,
0.820511285096538));
#17384=CARTESIAN_POINT('Ctrl Pts',(0.548874290046456,-0.159766064500479,
0.813159949759));
#17385=CARTESIAN_POINT('Ctrl Pts',(0.573915184558107,-0.190326085855194,
0.795684265985089));
#17386=CARTESIAN_POINT('Ctrl Pts',(0.587792702767295,-0.203463743702801,
0.78555112003688));
#17387=CARTESIAN_POINT('Ctrl Pts',(0.615966552324775,-0.224161999508995,
0.763642258217233));
#17388=CARTESIAN_POINT('Ctrl Pts',(0.631684198665438,-0.232861760990032,
0.750785745543687));
#17389=CARTESIAN_POINT('Ctrl Pts',(0.663382628119203,-0.244251601209411,
0.722929908501543));
#17390=CARTESIAN_POINT('Ctrl Pts',(0.679352081686668,-0.246942143572133,
0.707917883896095));
#17391=CARTESIAN_POINT('Ctrl Pts',(0.707917883896095,-0.246942143572133,
0.679352081686668));
#17392=CARTESIAN_POINT('Ctrl Pts',(0.722929908501543,-0.244251601209411,
0.663382628119203));
#17393=CARTESIAN_POINT('Ctrl Pts',(0.750785745543687,-0.232861760990032,
0.631684198665439));
#17394=CARTESIAN_POINT('Ctrl Pts',(0.763642258217232,-0.224161999508995,
0.615966552324775));
#17395=CARTESIAN_POINT('Ctrl Pts',(0.78555112003688,-0.203463743702801,
0.587792702767295));
#17396=CARTESIAN_POINT('Ctrl Pts',(0.795684265985088,-0.190326085855194,
0.573915184558108));
#17397=CARTESIAN_POINT('Ctrl Pts',(0.813159949759,-0.15976606450048,0.548874290046456));
#17398=CARTESIAN_POINT('Ctrl Pts',(0.820511285096538,-0.142345102874864,
0.537715343527944));
#17399=CARTESIAN_POINT('Ctrl Pts',(0.833661031856294,-0.099930567888331,
0.517157748491653));
#17400=CARTESIAN_POINT('Ctrl Pts',(0.838633903678357,-0.0740444353928835,
0.508899795931835));
#17401=CARTESIAN_POINT('Ctrl Pts',(0.841298510752801,-0.0476299999999999,
0.504455939115715));
#17402=CARTESIAN_POINT('',(0.528110872004958,-0.04763,0.871530771444223));
#17403=CARTESIAN_POINT('Origin',(0.707106781186547,-0.04763,0.707106781186548));
#17404=CARTESIAN_POINT('',(0.871530771444223,-0.04763,0.528110872004959));
#17405=CARTESIAN_POINT('Ctrl Pts',(0.871530771444223,-0.0476300000000001,
0.528110872004958));
#17406=CARTESIAN_POINT('Ctrl Pts',(0.87014664509073,-0.0609922781173483,
0.530395067942936));
#17407=CARTESIAN_POINT('Ctrl Pts',(0.868149331745851,-0.0742967091364493,
0.533674141594226));
#17408=CARTESIAN_POINT('Ctrl Pts',(0.85981294420286,-0.115492077056649,
0.54708917182331));
#17409=CARTESIAN_POINT('Ctrl Pts',(0.850993704737257,-0.141695629206859,
0.560922177770136));
#17410=CARTESIAN_POINT('Ctrl Pts',(0.830754510485543,-0.181890537957859,
0.590422647829571));
#17411=CARTESIAN_POINT('Ctrl Pts',(0.816896541396381,-0.201072148666545,
0.609616703125488));
#17412=CARTESIAN_POINT('Ctrl Pts',(0.792310597819928,-0.223955109275652,
0.641117951819998));
#17413=CARTESIAN_POINT('Ctrl Pts',(0.779109323683612,-0.232742381310829,
0.657208095763053));
#17414=CARTESIAN_POINT('Ctrl Pts',(0.750552691816206,-0.244234834628584,
0.68964083160521));
#17415=CARTESIAN_POINT('Ctrl Pts',(0.735185187071673,-0.246942143572133,
0.705971972091755));
#17416=CARTESIAN_POINT('Ctrl Pts',(0.705971972091754,-0.246942143572133,
0.735185187071673));
#17417=CARTESIAN_POINT('Ctrl Pts',(0.689640831605209,-0.244234834628584,
0.750552691816206));
#17418=CARTESIAN_POINT('Ctrl Pts',(0.657208095763052,-0.232742381310829,
0.779109323683612));
#17419=CARTESIAN_POINT('Ctrl Pts',(0.641117951819998,-0.223955109275652,
0.792310597819928));
#17420=CARTESIAN_POINT('Ctrl Pts',(0.609616703125487,-0.201072148666545,
0.816896541396382));
#17421=CARTESIAN_POINT('Ctrl Pts',(0.590422647829571,-0.181890537957858,
0.830754510485544));
#17422=CARTESIAN_POINT('Ctrl Pts',(0.560922177770135,-0.141695629206858,
0.850993704737257));
#17423=CARTESIAN_POINT('Ctrl Pts',(0.547089171823309,-0.115492077056649,
0.859812944202861));
#17424=CARTESIAN_POINT('Ctrl Pts',(0.533674141594226,-0.0742967091364491,
0.868149331745852));
#17425=CARTESIAN_POINT('Ctrl Pts',(0.530395067942936,-0.0609922781173483,
0.870146645090731));
#17426=CARTESIAN_POINT('Ctrl Pts',(0.528110872004958,-0.0476300000000001,
0.871530771444223));
#17427=CARTESIAN_POINT('Origin',(0.707106781186547,-0.04763,0.707106781186548));
#17428=CARTESIAN_POINT('Origin',(0.,-0.166705,0.));
#17429=CARTESIAN_POINT('',(0.242834539687906,-0.04763,0.989696097314));
#17430=CARTESIAN_POINT('Origin',(0.,-0.04763,0.));
#17431=CARTESIAN_POINT('',(-0.242834539687907,-0.04763,0.989696097314));
#17432=CARTESIAN_POINT('Ctrl Pts',(0.242834539687906,-0.04763,0.989696097314));
#17433=CARTESIAN_POINT('Ctrl Pts',(0.24024064412003,-0.0609922781173483,
0.990332542620729));
#17434=CARTESIAN_POINT('Ctrl Pts',(0.236509675094874,-0.0742967091364492,
0.991238884025248));
#17435=CARTESIAN_POINT('Ctrl Pts',(0.221129100087819,-0.115492077056649,
0.994830026707808));
#17436=CARTESIAN_POINT('Ctrl Pts',(0.205111543747588,-0.141695629206859,
0.998375294985966));
#17437=CARTESIAN_POINT('Ctrl Pts',(0.169940289819232,-0.181890537957859,
1.00492400591205));
#17438=CARTESIAN_POINT('Ctrl Pts',(0.1465689792446,-0.201072148666545,1.00869718865384));
#17439=CARTESIAN_POINT('Ctrl Pts',(0.106909345252087,-0.223955109275652,
1.01358704779679));
#17440=CARTESIAN_POINT('Ctrl Pts',(0.0861971848975941,-0.232742381310829,
1.0156297872271));
#17441=CARTESIAN_POINT('Ctrl Pts',(0.0430711894098822,-0.244234834628584,
1.01837060663223));
#17442=CARTESIAN_POINT('Ctrl Pts',(0.0206568624125605,-0.246942143572133,
1.019052));
#17443=CARTESIAN_POINT('Ctrl Pts',(-0.0206568624125608,-0.246942143572133,
1.019052));
#17444=CARTESIAN_POINT('Ctrl Pts',(-0.0430711894098825,-0.244234834628584,
1.01837060663223));
#17445=CARTESIAN_POINT('Ctrl Pts',(-0.0861971848975943,-0.232742381310829,
1.0156297872271));
#17446=CARTESIAN_POINT('Ctrl Pts',(-0.106909345252088,-0.223955109275652,
1.01358704779679));
#17447=CARTESIAN_POINT('Ctrl Pts',(-0.1465689792446,-0.201072148666545,
1.00869718865384));
#17448=CARTESIAN_POINT('Ctrl Pts',(-0.169940289819232,-0.181890537957859,
1.00492400591205));
#17449=CARTESIAN_POINT('Ctrl Pts',(-0.205111543747588,-0.141695629206859,
0.998375294985966));
#17450=CARTESIAN_POINT('Ctrl Pts',(-0.221129100087819,-0.115492077056649,
0.994830026707808));
#17451=CARTESIAN_POINT('Ctrl Pts',(-0.236509675094875,-0.0742967091364493,
0.991238884025248));
#17452=CARTESIAN_POINT('Ctrl Pts',(-0.24024064412003,-0.0609922781173483,
0.990332542620729));
#17453=CARTESIAN_POINT('Ctrl Pts',(-0.242834539687907,-0.04763,0.989696097314));
#17454=CARTESIAN_POINT('',(-0.528110872004959,-0.04763,0.871530771444223));
#17455=CARTESIAN_POINT('Origin',(0.,-0.04763,0.));
#17456=CARTESIAN_POINT('',(-0.871530771444223,-0.04763,0.528110872004958));
#17457=CARTESIAN_POINT('Ctrl Pts',(-0.528110872004958,-0.0476300000000001,
0.871530771444223));
#17458=CARTESIAN_POINT('Ctrl Pts',(-0.530395067942936,-0.0609922781173484,
0.87014664509073));
#17459=CARTESIAN_POINT('Ctrl Pts',(-0.533674141594226,-0.0742967091364493,
0.868149331745851));
#17460=CARTESIAN_POINT('Ctrl Pts',(-0.54708917182331,-0.115492077056649,
0.85981294420286));
#17461=CARTESIAN_POINT('Ctrl Pts',(-0.560922177770136,-0.141695629206859,
0.850993704737257));
#17462=CARTESIAN_POINT('Ctrl Pts',(-0.590422647829571,-0.181890537957859,
0.830754510485543));
#17463=CARTESIAN_POINT('Ctrl Pts',(-0.609616703125488,-0.201072148666545,
0.816896541396381));
#17464=CARTESIAN_POINT('Ctrl Pts',(-0.641117951819998,-0.223955109275652,
0.792310597819928));
#17465=CARTESIAN_POINT('Ctrl Pts',(-0.657208095763053,-0.232742381310829,
0.779109323683611));
#17466=CARTESIAN_POINT('Ctrl Pts',(-0.68964083160521,-0.244234834628584,
0.750552691816205));
#17467=CARTESIAN_POINT('Ctrl Pts',(-0.705971972091755,-0.246942143572133,
0.735185187071673));
#17468=CARTESIAN_POINT('Ctrl Pts',(-0.735185187071673,-0.246942143572133,
0.705971972091754));
#17469=CARTESIAN_POINT('Ctrl Pts',(-0.750552691816206,-0.244234834628584,
0.689640831605209));
#17470=CARTESIAN_POINT('Ctrl Pts',(-0.779109323683612,-0.232742381310829,
0.657208095763052));
#17471=CARTESIAN_POINT('Ctrl Pts',(-0.792310597819928,-0.223955109275652,
0.641117951819998));
#17472=CARTESIAN_POINT('Ctrl Pts',(-0.816896541396382,-0.201072148666545,
0.609616703125487));
#17473=CARTESIAN_POINT('Ctrl Pts',(-0.830754510485544,-0.181890537957858,
0.590422647829571));
#17474=CARTESIAN_POINT('Ctrl Pts',(-0.850993704737257,-0.141695629206858,
0.560922177770135));
#17475=CARTESIAN_POINT('Ctrl Pts',(-0.859812944202861,-0.115492077056649,
0.547089171823309));
#17476=CARTESIAN_POINT('Ctrl Pts',(-0.868149331745852,-0.0742967091364491,
0.533674141594226));
#17477=CARTESIAN_POINT('Ctrl Pts',(-0.870146645090731,-0.0609922781173483,
0.530395067942936));
#17478=CARTESIAN_POINT('Ctrl Pts',(-0.871530771444223,-0.04763,0.528110872004958));
#17479=CARTESIAN_POINT('',(-0.989696097314,-0.04763,0.242834539687906));
#17480=CARTESIAN_POINT('Origin',(0.,-0.04763,0.));
#17481=CARTESIAN_POINT('',(-1.019052,-0.246942143572133,1.248489836334E-16));
#17482=CARTESIAN_POINT('Ctrl Pts',(-0.989696097314,-0.04763,0.242834539687906));
#17483=CARTESIAN_POINT('Ctrl Pts',(-0.990332542620729,-0.0609922781173483,
0.24024064412003));
#17484=CARTESIAN_POINT('Ctrl Pts',(-0.991238884025248,-0.0742967091364492,
0.236509675094874));
#17485=CARTESIAN_POINT('Ctrl Pts',(-0.994830026707808,-0.115492077056649,
0.221129100087819));
#17486=CARTESIAN_POINT('Ctrl Pts',(-0.998375294985966,-0.141695629206859,
0.205111543747588));
#17487=CARTESIAN_POINT('Ctrl Pts',(-1.00492400591205,-0.181890537957859,
0.169940289819232));
#17488=CARTESIAN_POINT('Ctrl Pts',(-1.00869718865384,-0.201072148666545,
0.1465689792446));
#17489=CARTESIAN_POINT('Ctrl Pts',(-1.01358704779679,-0.223955109275652,
0.106909345252088));
#17490=CARTESIAN_POINT('Ctrl Pts',(-1.0156297872271,-0.232742381310829,
0.0861971848975944));
#17491=CARTESIAN_POINT('Ctrl Pts',(-1.01837060663223,-0.244234834628584,
0.0430711894098825));
#17492=CARTESIAN_POINT('Ctrl Pts',(-1.019052,-0.246942143572133,0.0206568624125608));
#17493=CARTESIAN_POINT('Ctrl Pts',(-1.019052,-0.246942143572133,1.2490009027033E-16));
#17494=CARTESIAN_POINT('',(-1.019052,-0.28578,1.24797876996471E-16));
#17495=CARTESIAN_POINT('',(-1.019052,-0.166705,1.24797876996471E-16));
#17496=CARTESIAN_POINT('Origin',(0.,-0.28578,0.));
#17497=CARTESIAN_POINT('',(-0.989696097314,-0.04763,-0.242834539687906));
#17498=CARTESIAN_POINT('Ctrl Pts',(-1.019052,-0.246942143572133,1.2490009027033E-16));
#17499=CARTESIAN_POINT('Ctrl Pts',(-1.019052,-0.246942143572133,-0.0206568624125605));
#17500=CARTESIAN_POINT('Ctrl Pts',(-1.01837060663223,-0.244234834628584,
-0.0430711894098822));
#17501=CARTESIAN_POINT('Ctrl Pts',(-1.0156297872271,-0.232742381310829,
-0.0861971848975941));
#17502=CARTESIAN_POINT('Ctrl Pts',(-1.01358704779679,-0.223955109275652,
-0.106909345252087));
#17503=CARTESIAN_POINT('Ctrl Pts',(-1.00869718865384,-0.201072148666546,
-0.1465689792446));
#17504=CARTESIAN_POINT('Ctrl Pts',(-1.00492400591205,-0.181890537957859,
-0.169940289819232));
#17505=CARTESIAN_POINT('Ctrl Pts',(-0.998375294985966,-0.141695629206859,
-0.205111543747588));
#17506=CARTESIAN_POINT('Ctrl Pts',(-0.994830026707808,-0.11549207705665,
-0.221129100087819));
#17507=CARTESIAN_POINT('Ctrl Pts',(-0.991238884025248,-0.0742967091364495,
-0.236509675094874));
#17508=CARTESIAN_POINT('Ctrl Pts',(-0.990332542620729,-0.0609922781173484,
-0.24024064412003));
#17509=CARTESIAN_POINT('Ctrl Pts',(-0.989696097314,-0.0476300000000001,
-0.242834539687907));
#17510=CARTESIAN_POINT('',(-0.871530771444223,-0.04763,-0.528110872004958));
#17511=CARTESIAN_POINT('Origin',(0.,-0.04763,0.));
#17512=CARTESIAN_POINT('',(-0.528110872004958,-0.04763,-0.871530771444223));
#17513=CARTESIAN_POINT('Ctrl Pts',(-0.871530771444223,-0.0476300000000001,
-0.528110872004958));
#17514=CARTESIAN_POINT('Ctrl Pts',(-0.87014664509073,-0.0609922781173484,
-0.530395067942936));
#17515=CARTESIAN_POINT('Ctrl Pts',(-0.868149331745851,-0.0742967091364494,
-0.533674141594226));
#17516=CARTESIAN_POINT('Ctrl Pts',(-0.85981294420286,-0.115492077056649,
-0.54708917182331));
#17517=CARTESIAN_POINT('Ctrl Pts',(-0.850993704737257,-0.141695629206859,
-0.560922177770136));
#17518=CARTESIAN_POINT('Ctrl Pts',(-0.830754510485543,-0.181890537957859,
-0.590422647829571));
#17519=CARTESIAN_POINT('Ctrl Pts',(-0.816896541396381,-0.201072148666546,
-0.609616703125488));
#17520=CARTESIAN_POINT('Ctrl Pts',(-0.792310597819928,-0.223955109275652,
-0.641117951819999));
#17521=CARTESIAN_POINT('Ctrl Pts',(-0.779109323683611,-0.232742381310829,
-0.657208095763053));
#17522=CARTESIAN_POINT('Ctrl Pts',(-0.750552691816205,-0.244234834628584,
-0.68964083160521));
#17523=CARTESIAN_POINT('Ctrl Pts',(-0.735185187071673,-0.246942143572133,
-0.705971972091755));
#17524=CARTESIAN_POINT('Ctrl Pts',(-0.705971972091754,-0.246942143572133,
-0.735185187071673));
#17525=CARTESIAN_POINT('Ctrl Pts',(-0.68964083160521,-0.244234834628584,
-0.750552691816206));
#17526=CARTESIAN_POINT('Ctrl Pts',(-0.657208095763052,-0.232742381310829,
-0.779109323683612));
#17527=CARTESIAN_POINT('Ctrl Pts',(-0.641117951819998,-0.223955109275652,
-0.792310597819928));
#17528=CARTESIAN_POINT('Ctrl Pts',(-0.609616703125488,-0.201072148666545,
-0.816896541396381));
#17529=CARTESIAN_POINT('Ctrl Pts',(-0.590422647829571,-0.181890537957859,
-0.830754510485543));
#17530=CARTESIAN_POINT('Ctrl Pts',(-0.560922177770136,-0.141695629206859,
-0.850993704737257));
#17531=CARTESIAN_POINT('Ctrl Pts',(-0.54708917182331,-0.115492077056649,
-0.85981294420286));
#17532=CARTESIAN_POINT('Ctrl Pts',(-0.533674141594226,-0.0742967091364494,
-0.868149331745852));
#17533=CARTESIAN_POINT('Ctrl Pts',(-0.530395067942936,-0.0609922781173484,
-0.870146645090731));
#17534=CARTESIAN_POINT('Ctrl Pts',(-0.528110872004958,-0.0476300000000001,
-0.871530771444223));
#17535=CARTESIAN_POINT('',(-0.242834539687906,-0.04763,-0.989696097314));
#17536=CARTESIAN_POINT('Origin',(0.,-0.04763,0.));
#17537=CARTESIAN_POINT('',(0.242834539687906,-0.04763,-0.989696097314));
#17538=CARTESIAN_POINT('Ctrl Pts',(-0.242834539687907,-0.04763,-0.989696097314));
#17539=CARTESIAN_POINT('Ctrl Pts',(-0.24024064412003,-0.0609922781173483,
-0.990332542620729));
#17540=CARTESIAN_POINT('Ctrl Pts',(-0.236509675094874,-0.0742967091364493,
-0.991238884025248));
#17541=CARTESIAN_POINT('Ctrl Pts',(-0.221129100087819,-0.115492077056649,
-0.994830026707808));
#17542=CARTESIAN_POINT('Ctrl Pts',(-0.205111543747588,-0.141695629206859,
-0.998375294985966));
#17543=CARTESIAN_POINT('Ctrl Pts',(-0.169940289819232,-0.181890537957859,
-1.00492400591205));
#17544=CARTESIAN_POINT('Ctrl Pts',(-0.1465689792446,-0.201072148666545,
-1.00869718865384));
#17545=CARTESIAN_POINT('Ctrl Pts',(-0.106909345252087,-0.223955109275652,
-1.01358704779679));
#17546=CARTESIAN_POINT('Ctrl Pts',(-0.0861971848975942,-0.232742381310829,
-1.0156297872271));
#17547=CARTESIAN_POINT('Ctrl Pts',(-0.0430711894098823,-0.244234834628584,
-1.01837060663223));
#17548=CARTESIAN_POINT('Ctrl Pts',(-0.0206568624125606,-0.246942143572133,
-1.019052));
#17549=CARTESIAN_POINT('Ctrl Pts',(0.0206568624125607,-0.246942143572133,
-1.019052));
#17550=CARTESIAN_POINT('Ctrl Pts',(0.0430711894098824,-0.244234834628584,
-1.01837060663223));
#17551=CARTESIAN_POINT('Ctrl Pts',(0.0861971848975943,-0.232742381310829,
-1.0156297872271));
#17552=CARTESIAN_POINT('Ctrl Pts',(0.106909345252088,-0.223955109275652,
-1.01358704779679));
#17553=CARTESIAN_POINT('Ctrl Pts',(0.1465689792446,-0.201072148666545,-1.00869718865384));
#17554=CARTESIAN_POINT('Ctrl Pts',(0.169940289819232,-0.181890537957859,
-1.00492400591205));
#17555=CARTESIAN_POINT('Ctrl Pts',(0.205111543747588,-0.141695629206859,
-0.998375294985966));
#17556=CARTESIAN_POINT('Ctrl Pts',(0.221129100087819,-0.115492077056649,
-0.994830026707808));
#17557=CARTESIAN_POINT('Ctrl Pts',(0.236509675094874,-0.0742967091364493,
-0.991238884025248));
#17558=CARTESIAN_POINT('Ctrl Pts',(0.24024064412003,-0.0609922781173484,
-0.990332542620729));
#17559=CARTESIAN_POINT('Ctrl Pts',(0.242834539687907,-0.04763,-0.989696097314));
#17560=CARTESIAN_POINT('',(0.528110872004958,-0.04763,-0.871530771444223));
#17561=CARTESIAN_POINT('Origin',(0.,-0.04763,0.));
#17562=CARTESIAN_POINT('',(0.871530771444223,-0.04763,-0.528110872004958));
#17563=CARTESIAN_POINT('Ctrl Pts',(0.528110872004958,-0.0476300000000001,
-0.871530771444223));
#17564=CARTESIAN_POINT('Ctrl Pts',(0.530395067942936,-0.0609922781173484,
-0.870146645090731));
#17565=CARTESIAN_POINT('Ctrl Pts',(0.533674141594226,-0.0742967091364493,
-0.868149331745851));
#17566=CARTESIAN_POINT('Ctrl Pts',(0.54708917182331,-0.115492077056649,
-0.85981294420286));
#17567=CARTESIAN_POINT('Ctrl Pts',(0.560922177770136,-0.141695629206859,
-0.850993704737257));
#17568=CARTESIAN_POINT('Ctrl Pts',(0.590422647829571,-0.181890537957859,
-0.830754510485543));
#17569=CARTESIAN_POINT('Ctrl Pts',(0.609616703125488,-0.201072148666545,
-0.816896541396381));
#17570=CARTESIAN_POINT('Ctrl Pts',(0.641117951819998,-0.223955109275652,
-0.792310597819928));
#17571=CARTESIAN_POINT('Ctrl Pts',(0.657208095763053,-0.232742381310829,
-0.779109323683612));
#17572=CARTESIAN_POINT('Ctrl Pts',(0.68964083160521,-0.244234834628584,
-0.750552691816206));
#17573=CARTESIAN_POINT('Ctrl Pts',(0.705971972091755,-0.246942143572133,
-0.735185187071673));
#17574=CARTESIAN_POINT('Ctrl Pts',(0.735185187071673,-0.246942143572133,
-0.705971972091754));
#17575=CARTESIAN_POINT('Ctrl Pts',(0.750552691816206,-0.244234834628584,
-0.68964083160521));
#17576=CARTESIAN_POINT('Ctrl Pts',(0.779109323683612,-0.232742381310829,
-0.657208095763053));
#17577=CARTESIAN_POINT('Ctrl Pts',(0.792310597819928,-0.223955109275652,
-0.641117951819998));
#17578=CARTESIAN_POINT('Ctrl Pts',(0.816896541396381,-0.201072148666545,
-0.609616703125488));
#17579=CARTESIAN_POINT('Ctrl Pts',(0.830754510485543,-0.181890537957859,
-0.590422647829571));
#17580=CARTESIAN_POINT('Ctrl Pts',(0.850993704737257,-0.141695629206859,
-0.560922177770136));
#17581=CARTESIAN_POINT('Ctrl Pts',(0.85981294420286,-0.115492077056649,
-0.54708917182331));
#17582=CARTESIAN_POINT('Ctrl Pts',(0.868149331745851,-0.0742967091364493,
-0.533674141594226));
#17583=CARTESIAN_POINT('Ctrl Pts',(0.870146645090731,-0.0609922781173484,
-0.530395067942936));
#17584=CARTESIAN_POINT('Ctrl Pts',(0.871530771444223,-0.0476300000000001,
-0.528110872004958));
#17585=CARTESIAN_POINT('',(0.989696097314,-0.04763,-0.242834539687906));
#17586=CARTESIAN_POINT('Origin',(0.,-0.04763,0.));
#17587=CARTESIAN_POINT('',(0.989696097314,-0.04763,0.242834539687906));
#17588=CARTESIAN_POINT('Ctrl Pts',(0.989696097314,-0.04763,-0.242834539687907));
#17589=CARTESIAN_POINT('Ctrl Pts',(0.990332542620729,-0.0609922781173483,
-0.24024064412003));
#17590=CARTESIAN_POINT('Ctrl Pts',(0.991238884025248,-0.0742967091364493,
-0.236509675094874));
#17591=CARTESIAN_POINT('Ctrl Pts',(0.994830026707808,-0.115492077056649,
-0.221129100087819));
#17592=CARTESIAN_POINT('Ctrl Pts',(0.998375294985966,-0.141695629206859,
-0.205111543747588));
#17593=CARTESIAN_POINT('Ctrl Pts',(1.00492400591205,-0.181890537957859,
-0.169940289819232));
#17594=CARTESIAN_POINT('Ctrl Pts',(1.00869718865384,-0.201072148666545,
-0.1465689792446));
#17595=CARTESIAN_POINT('Ctrl Pts',(1.01358704779679,-0.223955109275652,
-0.106909345252087));
#17596=CARTESIAN_POINT('Ctrl Pts',(1.0156297872271,-0.232742381310829,-0.0861971848975942));
#17597=CARTESIAN_POINT('Ctrl Pts',(1.01837060663223,-0.244234834628584,
-0.0430711894098823));
#17598=CARTESIAN_POINT('Ctrl Pts',(1.019052,-0.246942143572133,-0.0206568624125607));
#17599=CARTESIAN_POINT('Ctrl Pts',(1.019052,-0.246942143572133,0.0206568624125607));
#17600=CARTESIAN_POINT('Ctrl Pts',(1.01837060663223,-0.244234834628584,
0.0430711894098823));
#17601=CARTESIAN_POINT('Ctrl Pts',(1.0156297872271,-0.232742381310829,0.0861971848975942));
#17602=CARTESIAN_POINT('Ctrl Pts',(1.01358704779679,-0.223955109275652,
0.106909345252087));
#17603=CARTESIAN_POINT('Ctrl Pts',(1.00869718865384,-0.201072148666545,
0.1465689792446));
#17604=CARTESIAN_POINT('Ctrl Pts',(1.00492400591205,-0.181890537957859,
0.169940289819232));
#17605=CARTESIAN_POINT('Ctrl Pts',(0.998375294985966,-0.141695629206859,
0.205111543747588));
#17606=CARTESIAN_POINT('Ctrl Pts',(0.994830026707808,-0.115492077056649,
0.221129100087819));
#17607=CARTESIAN_POINT('Ctrl Pts',(0.991238884025248,-0.0742967091364492,
0.236509675094874));
#17608=CARTESIAN_POINT('Ctrl Pts',(0.990332542620729,-0.0609922781173483,
0.24024064412003));
#17609=CARTESIAN_POINT('Ctrl Pts',(0.989696097314,-0.04763,0.242834539687907));
#17610=CARTESIAN_POINT('Origin',(0.,-0.04763,0.));
#17611=CARTESIAN_POINT('Origin',(0.,-0.04763,0.));
#17612=CARTESIAN_POINT('',(0.238183666596899,-0.04763,0.951592097314));
#17613=CARTESIAN_POINT('Origin',(0.,-0.04763,0.));
#17614=CARTESIAN_POINT('Origin',(-1.94289029309402E-16,-0.04763,1.));
#17615=CARTESIAN_POINT('Origin',(-1.94289029309402E-16,0.,1.));
#17616=CARTESIAN_POINT('',(-0.2381836665969,-0.04763,0.951592097314));
#17617=CARTESIAN_POINT('Ctrl Pts',(-0.238183666596899,-0.0476299999999999,
0.951592097314));
#17618=CARTESIAN_POINT('Ctrl Pts',(-0.233157223576062,-0.0740444353928835,
0.952850216871763));
#17619=CARTESIAN_POINT('Ctrl Pts',(-0.223801617934946,-0.0999305678883309,
0.955173119738174));
#17620=CARTESIAN_POINT('Ctrl Pts',(-0.199966927975188,-0.142345102874864,
0.960411259488514));
#17621=CARTESIAN_POINT('Ctrl Pts',(-0.1868781821531,-0.159766064500479,
0.963103647174702));
#17622=CARTESIAN_POINT('Ctrl Pts',(-0.15681442133453,-0.190326085855194,
0.968453058988463));
#17623=CARTESIAN_POINT('Ctrl Pts',(-0.139836317888043,-0.203463743702801,
0.971100730005489));
#17624=CARTESIAN_POINT('Ctrl Pts',(-0.104422493053067,-0.224161999508995,
0.975530745318961));
#17625=CARTESIAN_POINT('Ctrl Pts',(-0.0842175114474176,-0.232861760990032,
0.977553872336861));
#17626=CARTESIAN_POINT('Ctrl Pts',(-0.0421062857595701,-0.244251601209411,
0.980270995488453));
#17627=CARTESIAN_POINT('Ctrl Pts',(-0.0201990724523197,-0.246942143572133,
0.980948));
#17628=CARTESIAN_POINT('Ctrl Pts',(0.020199072452319,-0.246942143572133,
0.980948));
#17629=CARTESIAN_POINT('Ctrl Pts',(0.0421062857595694,-0.244251601209411,
0.980270995488454));
#17630=CARTESIAN_POINT('Ctrl Pts',(0.0842175114474169,-0.232861760990032,
0.977553872336861));
#17631=CARTESIAN_POINT('Ctrl Pts',(0.104422493053067,-0.224161999508995,
0.975530745318961));
#17632=CARTESIAN_POINT('Ctrl Pts',(0.139836317888042,-0.203463743702801,
0.971100730005489));
#17633=CARTESIAN_POINT('Ctrl Pts',(0.15681442133453,-0.190326085855194,
0.968453058988463));
#17634=CARTESIAN_POINT('Ctrl Pts',(0.1868781821531,-0.15976606450048,0.963103647174702));
#17635=CARTESIAN_POINT('Ctrl Pts',(0.199966927975188,-0.142345102874864,
0.960411259488514));
#17636=CARTESIAN_POINT('Ctrl Pts',(0.223801617934945,-0.0999305678883309,
0.955173119738174));
#17637=CARTESIAN_POINT('Ctrl Pts',(0.233157223576061,-0.0740444353928835,
0.952850216871763));
#17638=CARTESIAN_POINT('Ctrl Pts',(0.238183666596899,-0.0476299999999999,
0.951592097314));
#17639=CARTESIAN_POINT('Origin',(-1.94289029309402E-16,-0.04763,1.));
#17640=CARTESIAN_POINT('Origin',(0.,-0.04763,0.));
#17641=CARTESIAN_POINT('',(-0.504455939115715,-0.04763,0.841298510752802));
#17642=CARTESIAN_POINT('Origin',(0.,-0.04763,0.));
#17643=CARTESIAN_POINT('Origin',(-0.707106781186548,-0.04763,0.707106781186547));
#17644=CARTESIAN_POINT('Origin',(-0.707106781186548,0.,0.707106781186547));
#17645=CARTESIAN_POINT('',(-0.841298510752802,-0.04763,0.504455939115715));
#17646=CARTESIAN_POINT('Ctrl Pts',(-0.841298510752802,-0.04763,0.504455939115715));
#17647=CARTESIAN_POINT('Ctrl Pts',(-0.838633903678357,-0.0740444353928835,
0.508899795931835));
#17648=CARTESIAN_POINT('Ctrl Pts',(-0.833661031856294,-0.0999305678883309,
0.517157748491652));
#17649=CARTESIAN_POINT('Ctrl Pts',(-0.820511285096538,-0.142345102874864,
0.537715343527944));
#17650=CARTESIAN_POINT('Ctrl Pts',(-0.813159949759,-0.159766064500479,0.548874290046456));
#17651=CARTESIAN_POINT('Ctrl Pts',(-0.795684265985089,-0.190326085855194,
0.573915184558107));
#17652=CARTESIAN_POINT('Ctrl Pts',(-0.78555112003688,-0.203463743702801,
0.587792702767295));
#17653=CARTESIAN_POINT('Ctrl Pts',(-0.763642258217233,-0.224161999508995,
0.615966552324775));
#17654=CARTESIAN_POINT('Ctrl Pts',(-0.750785745543687,-0.232861760990032,
0.631684198665438));
#17655=CARTESIAN_POINT('Ctrl Pts',(-0.722929908501543,-0.244251601209411,
0.663382628119203));
#17656=CARTESIAN_POINT('Ctrl Pts',(-0.707917883896095,-0.246942143572133,
0.679352081686668));
#17657=CARTESIAN_POINT('Ctrl Pts',(-0.679352081686668,-0.246942143572133,
0.707917883896095));
#17658=CARTESIAN_POINT('Ctrl Pts',(-0.663382628119203,-0.244251601209411,
0.722929908501544));
#17659=CARTESIAN_POINT('Ctrl Pts',(-0.631684198665438,-0.232861760990031,
0.750785745543687));
#17660=CARTESIAN_POINT('Ctrl Pts',(-0.615966552324775,-0.224161999508995,
0.763642258217233));
#17661=CARTESIAN_POINT('Ctrl Pts',(-0.587792702767295,-0.203463743702801,
0.78555112003688));
#17662=CARTESIAN_POINT('Ctrl Pts',(-0.573915184558107,-0.190326085855194,
0.795684265985088));
#17663=CARTESIAN_POINT('Ctrl Pts',(-0.548874290046456,-0.159766064500479,
0.813159949759));
#17664=CARTESIAN_POINT('Ctrl Pts',(-0.537715343527944,-0.142345102874864,
0.820511285096538));
#17665=CARTESIAN_POINT('Ctrl Pts',(-0.517157748491652,-0.0999305678883309,
0.833661031856294));
#17666=CARTESIAN_POINT('Ctrl Pts',(-0.508899795931835,-0.0740444353928835,
0.838633903678357));
#17667=CARTESIAN_POINT('Ctrl Pts',(-0.504455939115716,-0.04763,0.841298510752801));
#17668=CARTESIAN_POINT('Origin',(-0.707106781186548,-0.04763,0.707106781186547));
#17669=CARTESIAN_POINT('Origin',(0.,-0.04763,0.));
#17670=CARTESIAN_POINT('',(-0.951592097314,-0.04763,0.238183666596899));
#17671=CARTESIAN_POINT('Origin',(0.,-0.04763,0.));
#17672=CARTESIAN_POINT('Origin',(-1.,-0.04763,-1.11022302462516E-16));
#17673=CARTESIAN_POINT('Origin',(-1.,0.,-1.11022302462516E-16));
#17674=CARTESIAN_POINT('',(-0.951592097314,-0.04763,-0.2381836665969));
#17675=CARTESIAN_POINT('',(-0.980948,-0.246942143572133,1.08514323328844E-18));
#17676=CARTESIAN_POINT('Ctrl Pts',(-0.951592097314,-0.04763,-0.238183666596899));
#17677=CARTESIAN_POINT('Ctrl Pts',(-0.952850216871763,-0.0740444353928835,
-0.233157223576062));
#17678=CARTESIAN_POINT('Ctrl Pts',(-0.955173119738174,-0.0999305678883309,
-0.223801617934946));
#17679=CARTESIAN_POINT('Ctrl Pts',(-0.960411259488514,-0.142345102874864,
-0.199966927975188));
#17680=CARTESIAN_POINT('Ctrl Pts',(-0.963103647174702,-0.159766064500479,
-0.1868781821531));
#17681=CARTESIAN_POINT('Ctrl Pts',(-0.968453058988463,-0.190326085855194,
-0.15681442133453));
#17682=CARTESIAN_POINT('Ctrl Pts',(-0.971100730005489,-0.203463743702801,
-0.139836317888043));
#17683=CARTESIAN_POINT('Ctrl Pts',(-0.975530745318961,-0.224161999508995,
-0.104422493053067));
#17684=CARTESIAN_POINT('Ctrl Pts',(-0.977553872336861,-0.232861760990032,
-0.0842175114474175));
#17685=CARTESIAN_POINT('Ctrl Pts',(-0.980270995488453,-0.244251601209411,
-0.0421062857595699));
#17686=CARTESIAN_POINT('Ctrl Pts',(-0.980948,-0.246942143572133,-0.0201990724523195));
#17687=CARTESIAN_POINT('Ctrl Pts',(-0.980948,-0.246942143572133,-1.17961196366423E-16));
#17688=CARTESIAN_POINT('Origin',(-1.,-0.04763,-1.11022302462516E-16));
#17689=CARTESIAN_POINT('Ctrl Pts',(-0.980948,-0.246942143572133,-1.17961196366423E-16));
#17690=CARTESIAN_POINT('Ctrl Pts',(-0.980948,-0.246942143572133,0.0201990724523192));
#17691=CARTESIAN_POINT('Ctrl Pts',(-0.980270995488453,-0.244251601209411,
0.0421062857595695));
#17692=CARTESIAN_POINT('Ctrl Pts',(-0.977553872336861,-0.232861760990032,
0.0842175114474169));
#17693=CARTESIAN_POINT('Ctrl Pts',(-0.975530745318961,-0.224161999508995,
0.104422493053066));
#17694=CARTESIAN_POINT('Ctrl Pts',(-0.971100730005489,-0.203463743702801,
0.139836317888042));
#17695=CARTESIAN_POINT('Ctrl Pts',(-0.968453058988463,-0.190326085855194,
0.15681442133453));
#17696=CARTESIAN_POINT('Ctrl Pts',(-0.963103647174702,-0.15976606450048,
0.1868781821531));
#17697=CARTESIAN_POINT('Ctrl Pts',(-0.960411259488514,-0.142345102874864,
0.199966927975188));
#17698=CARTESIAN_POINT('Ctrl Pts',(-0.955173119738174,-0.099930567888331,
0.223801617934945));
#17699=CARTESIAN_POINT('Ctrl Pts',(-0.952850216871763,-0.0740444353928835,
0.233157223576061));
#17700=CARTESIAN_POINT('Ctrl Pts',(-0.951592097314,-0.04763,0.238183666596899));
#17701=CARTESIAN_POINT('Origin',(0.,-0.04763,0.));
#17702=CARTESIAN_POINT('',(-0.841298510752802,-0.04763,-0.504455939115715));
#17703=CARTESIAN_POINT('Origin',(0.,-0.04763,0.));
#17704=CARTESIAN_POINT('Origin',(-0.707106781186547,-0.04763,-0.707106781186548));
#17705=CARTESIAN_POINT('Origin',(-0.707106781186547,0.,-0.707106781186548));
#17706=CARTESIAN_POINT('',(-0.504455939115715,-0.04763,-0.841298510752802));
#17707=CARTESIAN_POINT('Ctrl Pts',(-0.504455939115715,-0.04763,-0.841298510752802));
#17708=CARTESIAN_POINT('Ctrl Pts',(-0.508899795931835,-0.0740444353928835,
-0.838633903678357));
#17709=CARTESIAN_POINT('Ctrl Pts',(-0.517157748491652,-0.0999305678883309,
-0.833661031856294));
#17710=CARTESIAN_POINT('Ctrl Pts',(-0.537715343527944,-0.142345102874864,
-0.820511285096538));
#17711=CARTESIAN_POINT('Ctrl Pts',(-0.548874290046456,-0.159766064500479,
-0.813159949759));
#17712=CARTESIAN_POINT('Ctrl Pts',(-0.573915184558107,-0.190326085855194,
-0.795684265985089));
#17713=CARTESIAN_POINT('Ctrl Pts',(-0.587792702767295,-0.203463743702801,
-0.78555112003688));
#17714=CARTESIAN_POINT('Ctrl Pts',(-0.615966552324775,-0.224161999508995,
-0.763642258217233));
#17715=CARTESIAN_POINT('Ctrl Pts',(-0.631684198665438,-0.232861760990032,
-0.750785745543687));
#17716=CARTESIAN_POINT('Ctrl Pts',(-0.663382628119203,-0.244251601209411,
-0.722929908501543));
#17717=CARTESIAN_POINT('Ctrl Pts',(-0.679352081686668,-0.246942143572133,
-0.707917883896095));
#17718=CARTESIAN_POINT('Ctrl Pts',(-0.707917883896095,-0.246942143572133,
-0.679352081686668));
#17719=CARTESIAN_POINT('Ctrl Pts',(-0.722929908501543,-0.244251601209411,
-0.663382628119203));
#17720=CARTESIAN_POINT('Ctrl Pts',(-0.750785745543687,-0.232861760990032,
-0.631684198665439));
#17721=CARTESIAN_POINT('Ctrl Pts',(-0.763642258217232,-0.224161999508995,
-0.615966552324775));
#17722=CARTESIAN_POINT('Ctrl Pts',(-0.78555112003688,-0.203463743702801,
-0.587792702767295));
#17723=CARTESIAN_POINT('Ctrl Pts',(-0.795684265985088,-0.190326085855194,
-0.573915184558107));
#17724=CARTESIAN_POINT('Ctrl Pts',(-0.813159949759,-0.15976606450048,-0.548874290046456));
#17725=CARTESIAN_POINT('Ctrl Pts',(-0.820511285096538,-0.142345102874864,
-0.537715343527944));
#17726=CARTESIAN_POINT('Ctrl Pts',(-0.833661031856294,-0.0999305678883311,
-0.517157748491652));
#17727=CARTESIAN_POINT('Ctrl Pts',(-0.838633903678357,-0.0740444353928836,
-0.508899795931835));
#17728=CARTESIAN_POINT('Ctrl Pts',(-0.841298510752801,-0.04763,-0.504455939115715));
#17729=CARTESIAN_POINT('Origin',(-0.707106781186547,-0.04763,-0.707106781186548));
#17730=CARTESIAN_POINT('Origin',(0.,-0.04763,0.));
#17731=CARTESIAN_POINT('',(-0.238183666596899,-0.04763,-0.951592097314));
#17732=CARTESIAN_POINT('Origin',(0.,-0.04763,0.));
#17733=CARTESIAN_POINT('Origin',(5.55111512312578E-17,-0.04763,-1.));
#17734=CARTESIAN_POINT('Origin',(5.55111512312578E-17,0.,-1.));
#17735=CARTESIAN_POINT('',(0.238183666596899,-0.04763,-0.951592097314));
#17736=CARTESIAN_POINT('Ctrl Pts',(0.238183666596899,-0.04763,-0.951592097314));
#17737=CARTESIAN_POINT('Ctrl Pts',(0.233157223576062,-0.0740444353928835,
-0.952850216871763));
#17738=CARTESIAN_POINT('Ctrl Pts',(0.223801617934946,-0.099930567888331,
-0.955173119738174));
#17739=CARTESIAN_POINT('Ctrl Pts',(0.199966927975188,-0.142345102874864,
-0.960411259488514));
#17740=CARTESIAN_POINT('Ctrl Pts',(0.1868781821531,-0.15976606450048,-0.963103647174702));
#17741=CARTESIAN_POINT('Ctrl Pts',(0.15681442133453,-0.190326085855194,
-0.968453058988463));
#17742=CARTESIAN_POINT('Ctrl Pts',(0.139836317888042,-0.203463743702801,
-0.971100730005489));
#17743=CARTESIAN_POINT('Ctrl Pts',(0.104422493053067,-0.224161999508995,
-0.975530745318961));
#17744=CARTESIAN_POINT('Ctrl Pts',(0.0842175114474173,-0.232861760990032,
-0.977553872336861));
#17745=CARTESIAN_POINT('Ctrl Pts',(0.0421062857595698,-0.244251601209411,
-0.980270995488453));
#17746=CARTESIAN_POINT('Ctrl Pts',(0.0201990724523194,-0.246942143572133,
-0.980948));
#17747=CARTESIAN_POINT('Ctrl Pts',(-0.0201990724523193,-0.246942143572133,
-0.980948));
#17748=CARTESIAN_POINT('Ctrl Pts',(-0.0421062857595697,-0.244251601209411,
-0.980270995488453));
#17749=CARTESIAN_POINT('Ctrl Pts',(-0.0842175114474171,-0.232861760990032,
-0.977553872336861));
#17750=CARTESIAN_POINT('Ctrl Pts',(-0.104422493053067,-0.224161999508995,
-0.975530745318961));
#17751=CARTESIAN_POINT('Ctrl Pts',(-0.139836317888042,-0.203463743702801,
-0.971100730005489));
#17752=CARTESIAN_POINT('Ctrl Pts',(-0.15681442133453,-0.190326085855194,
-0.968453058988463));
#17753=CARTESIAN_POINT('Ctrl Pts',(-0.1868781821531,-0.15976606450048,-0.963103647174702));
#17754=CARTESIAN_POINT('Ctrl Pts',(-0.199966927975188,-0.142345102874864,
-0.960411259488514));
#17755=CARTESIAN_POINT('Ctrl Pts',(-0.223801617934945,-0.099930567888331,
-0.955173119738174));
#17756=CARTESIAN_POINT('Ctrl Pts',(-0.233157223576062,-0.0740444353928835,
-0.952850216871763));
#17757=CARTESIAN_POINT('Ctrl Pts',(-0.238183666596899,-0.0476299999999999,
-0.951592097314));
#17758=CARTESIAN_POINT('Origin',(5.55111512312578E-17,-0.04763,-1.));
#17759=CARTESIAN_POINT('Origin',(0.,-0.04763,0.));
#17760=CARTESIAN_POINT('',(0.504455939115715,-0.04763,-0.841298510752802));
#17761=CARTESIAN_POINT('Origin',(0.,-0.04763,0.));
#17762=CARTESIAN_POINT('Origin',(0.707106781186548,-0.04763,-0.707106781186547));
#17763=CARTESIAN_POINT('Origin',(0.707106781186548,0.,-0.707106781186547));
#17764=CARTESIAN_POINT('',(0.841298510752802,-0.04763,-0.504455939115715));
#17765=CARTESIAN_POINT('Ctrl Pts',(0.841298510752802,-0.04763,-0.504455939115715));
#17766=CARTESIAN_POINT('Ctrl Pts',(0.838633903678357,-0.0740444353928835,
-0.508899795931835));
#17767=CARTESIAN_POINT('Ctrl Pts',(0.833661031856294,-0.0999305678883309,
-0.517157748491652));
#17768=CARTESIAN_POINT('Ctrl Pts',(0.820511285096538,-0.142345102874864,
-0.537715343527944));
#17769=CARTESIAN_POINT('Ctrl Pts',(0.813159949759,-0.159766064500479,-0.548874290046456));
#17770=CARTESIAN_POINT('Ctrl Pts',(0.795684265985088,-0.190326085855194,
-0.573915184558107));
#17771=CARTESIAN_POINT('Ctrl Pts',(0.78555112003688,-0.203463743702801,
-0.587792702767295));
#17772=CARTESIAN_POINT('Ctrl Pts',(0.763642258217233,-0.224161999508995,
-0.615966552324775));
#17773=CARTESIAN_POINT('Ctrl Pts',(0.750785745543687,-0.232861760990032,
-0.631684198665438));
#17774=CARTESIAN_POINT('Ctrl Pts',(0.722929908501543,-0.244251601209411,
-0.663382628119203));
#17775=CARTESIAN_POINT('Ctrl Pts',(0.707917883896095,-0.246942143572133,
-0.679352081686668));
#17776=CARTESIAN_POINT('Ctrl Pts',(0.679352081686668,-0.246942143572133,
-0.707917883896095));
#17777=CARTESIAN_POINT('Ctrl Pts',(0.663382628119203,-0.244251601209411,
-0.722929908501543));
#17778=CARTESIAN_POINT('Ctrl Pts',(0.631684198665438,-0.232861760990032,
-0.750785745543687));
#17779=CARTESIAN_POINT('Ctrl Pts',(0.615966552324775,-0.224161999508995,
-0.763642258217232));
#17780=CARTESIAN_POINT('Ctrl Pts',(0.587792702767295,-0.203463743702801,
-0.78555112003688));
#17781=CARTESIAN_POINT('Ctrl Pts',(0.573915184558107,-0.190326085855194,
-0.795684265985088));
#17782=CARTESIAN_POINT('Ctrl Pts',(0.548874290046456,-0.159766064500479,
-0.813159949759));
#17783=CARTESIAN_POINT('Ctrl Pts',(0.537715343527944,-0.142345102874864,
-0.820511285096538));
#17784=CARTESIAN_POINT('Ctrl Pts',(0.517157748491652,-0.099930567888331,
-0.833661031856294));
#17785=CARTESIAN_POINT('Ctrl Pts',(0.508899795931835,-0.0740444353928835,
-0.838633903678357));
#17786=CARTESIAN_POINT('Ctrl Pts',(0.504455939115715,-0.04763,-0.841298510752801));
#17787=CARTESIAN_POINT('Origin',(0.707106781186548,-0.04763,-0.707106781186547));
#17788=CARTESIAN_POINT('Origin',(0.,-0.166705,0.));
#17789=CARTESIAN_POINT('',(-0.980948,-0.28578,1.20131482833E-16));
#17790=CARTESIAN_POINT('Origin',(0.,-0.28578,0.));
#17791=CARTESIAN_POINT('',(-0.980948,-0.166705,1.20131482833E-16));
#17792=CARTESIAN_POINT('',(0.951592097314,-0.04763,0.238183666596899));
#17793=CARTESIAN_POINT('Origin',(0.,-0.04763,0.));
#17794=CARTESIAN_POINT('',(0.951592097314,-0.04763,-0.238183666596899));
#17795=CARTESIAN_POINT('Ctrl Pts',(0.951592097314,-0.04763,0.238183666596899));
#17796=CARTESIAN_POINT('Ctrl Pts',(0.952850216871763,-0.0740444353928835,
0.233157223576062));
#17797=CARTESIAN_POINT('Ctrl Pts',(0.955173119738174,-0.099930567888331,
0.223801617934945));
#17798=CARTESIAN_POINT('Ctrl Pts',(0.960411259488514,-0.142345102874864,
0.199966927975188));
#17799=CARTESIAN_POINT('Ctrl Pts',(0.963103647174702,-0.15976606450048,
0.1868781821531));
#17800=CARTESIAN_POINT('Ctrl Pts',(0.968453058988463,-0.190326085855194,
0.15681442133453));
#17801=CARTESIAN_POINT('Ctrl Pts',(0.971100730005489,-0.203463743702801,
0.139836317888042));
#17802=CARTESIAN_POINT('Ctrl Pts',(0.975530745318961,-0.224161999508995,
0.104422493053067));
#17803=CARTESIAN_POINT('Ctrl Pts',(0.977553872336861,-0.232861760990032,
0.0842175114474172));
#17804=CARTESIAN_POINT('Ctrl Pts',(0.980270995488453,-0.244251601209411,
0.0421062857595697));
#17805=CARTESIAN_POINT('Ctrl Pts',(0.980948,-0.246942143572133,0.0201990724523194));
#17806=CARTESIAN_POINT('Ctrl Pts',(0.980948,-0.246942143572133,-0.0201990724523194));
#17807=CARTESIAN_POINT('Ctrl Pts',(0.980270995488453,-0.244251601209411,
-0.0421062857595697));
#17808=CARTESIAN_POINT('Ctrl Pts',(0.977553872336861,-0.232861760990032,
-0.0842175114474172));
#17809=CARTESIAN_POINT('Ctrl Pts',(0.975530745318961,-0.224161999508995,
-0.104422493053067));
#17810=CARTESIAN_POINT('Ctrl Pts',(0.971100730005489,-0.203463743702801,
-0.139836317888042));
#17811=CARTESIAN_POINT('Ctrl Pts',(0.968453058988463,-0.190326085855194,
-0.15681442133453));
#17812=CARTESIAN_POINT('Ctrl Pts',(0.963103647174702,-0.15976606450048,
-0.1868781821531));
#17813=CARTESIAN_POINT('Ctrl Pts',(0.960411259488514,-0.142345102874864,
-0.199966927975188));
#17814=CARTESIAN_POINT('Ctrl Pts',(0.955173119738174,-0.099930567888331,
-0.223801617934945));
#17815=CARTESIAN_POINT('Ctrl Pts',(0.952850216871763,-0.0740444353928835,
-0.233157223576062));
#17816=CARTESIAN_POINT('Ctrl Pts',(0.951592097314,-0.0476299999999999,-0.238183666596899));
#17817=CARTESIAN_POINT('Origin',(0.,-0.04763,0.));
#17818=CARTESIAN_POINT('Origin',(0.,-0.04763,0.));
#17819=CARTESIAN_POINT('Origin',(1.,-0.04763,0.));
#17820=CARTESIAN_POINT('Origin',(1.,0.,0.));
#17821=CARTESIAN_POINT('Origin',(1.,-0.04763,0.));
#17822=CARTESIAN_POINT('Origin',(0.,-0.28578,0.));
#17823=CARTESIAN_POINT('Origin',(0.,-0.04763,0.));
#20009=UNCERTAINTY_MEASURE_WITH_UNIT(LENGTH_MEASURE(0.001),#20097,
'DISTANCE_ACCURACY_VALUE',
'Maximum model space distance between geometric entities at asserted c
onnectivities');
#20042=UNCERTAINTY_MEASURE_WITH_UNIT(LENGTH_MEASURE(0.001),#20097,
'DISTANCE_ACCURACY_VALUE',
'Maximum model space distance between geometric entities at asserted c
onnectivities');
#20063=(
GEOMETRIC_REPRESENTATION_CONTEXT(3)
GLOBAL_UNCERTAINTY_ASSIGNED_CONTEXT((#20009))
GLOBAL_UNIT_ASSIGNED_CONTEXT((#20097,#20099,#20100))
REPRESENTATION_CONTEXT('','3D')
);
#20096=(
GEOMETRIC_REPRESENTATION_CONTEXT(3)
GLOBAL_UNCERTAINTY_ASSIGNED_CONTEXT((#20042))
GLOBAL_UNIT_ASSIGNED_CONTEXT((#20097,#20099,#20100))
REPRESENTATION_CONTEXT('','3D')
);
#20097=(
LENGTH_UNIT()
NAMED_UNIT(*)
SI_UNIT(.CENTI.,.METRE.)
);
#20099=(
NAMED_UNIT(*)
PLANE_ANGLE_UNIT()
SI_UNIT($,.RADIAN.)
);
#20100=(
NAMED_UNIT(*)
SI_UNIT($,.STERADIAN.)
SOLID_ANGLE_UNIT()
);
#20121=SHAPE_DEFINITION_REPRESENTATION(#20174,#20332);
#20174=PRODUCT_DEFINITION_SHAPE('',$,#20386);
#20332=SHAPE_REPRESENTATION('',(#11974),#20063);
#20365=PRODUCT_DEFINITION_CONTEXT('part definition',#20526,'design');
#20386=PRODUCT_DEFINITION('Cage','Cage',#20439,#20365);
#20439=PRODUCT_DEFINITION_FORMATION('',$,#20548);
#20526=APPLICATION_CONTEXT(
'Core Data for Automotive Mechanical Design Process');
#20527=PRODUCT_CONTEXT('part definition',#20526,'mechanical');
#20548=PRODUCT('Cage','Cage','Cage',(#20527));
#20644=COLOUR_RGB('Grey',0.48,0.52,0.57);
#20645=FILL_AREA_STYLE_COLOUR('',#20644);
#20646=FILL_AREA_STYLE('',(#20645));
#20647=SURFACE_STYLE_FILL_AREA(#20646);
#20648=SURFACE_SIDE_STYLE('',(#20647));
#20649=SURFACE_STYLE_USAGE(.BOTH.,#20648);
#20650=PRESENTATION_STYLE_ASSIGNMENT((#20649));
ENDSEC;
END-ISO-10303-21;
